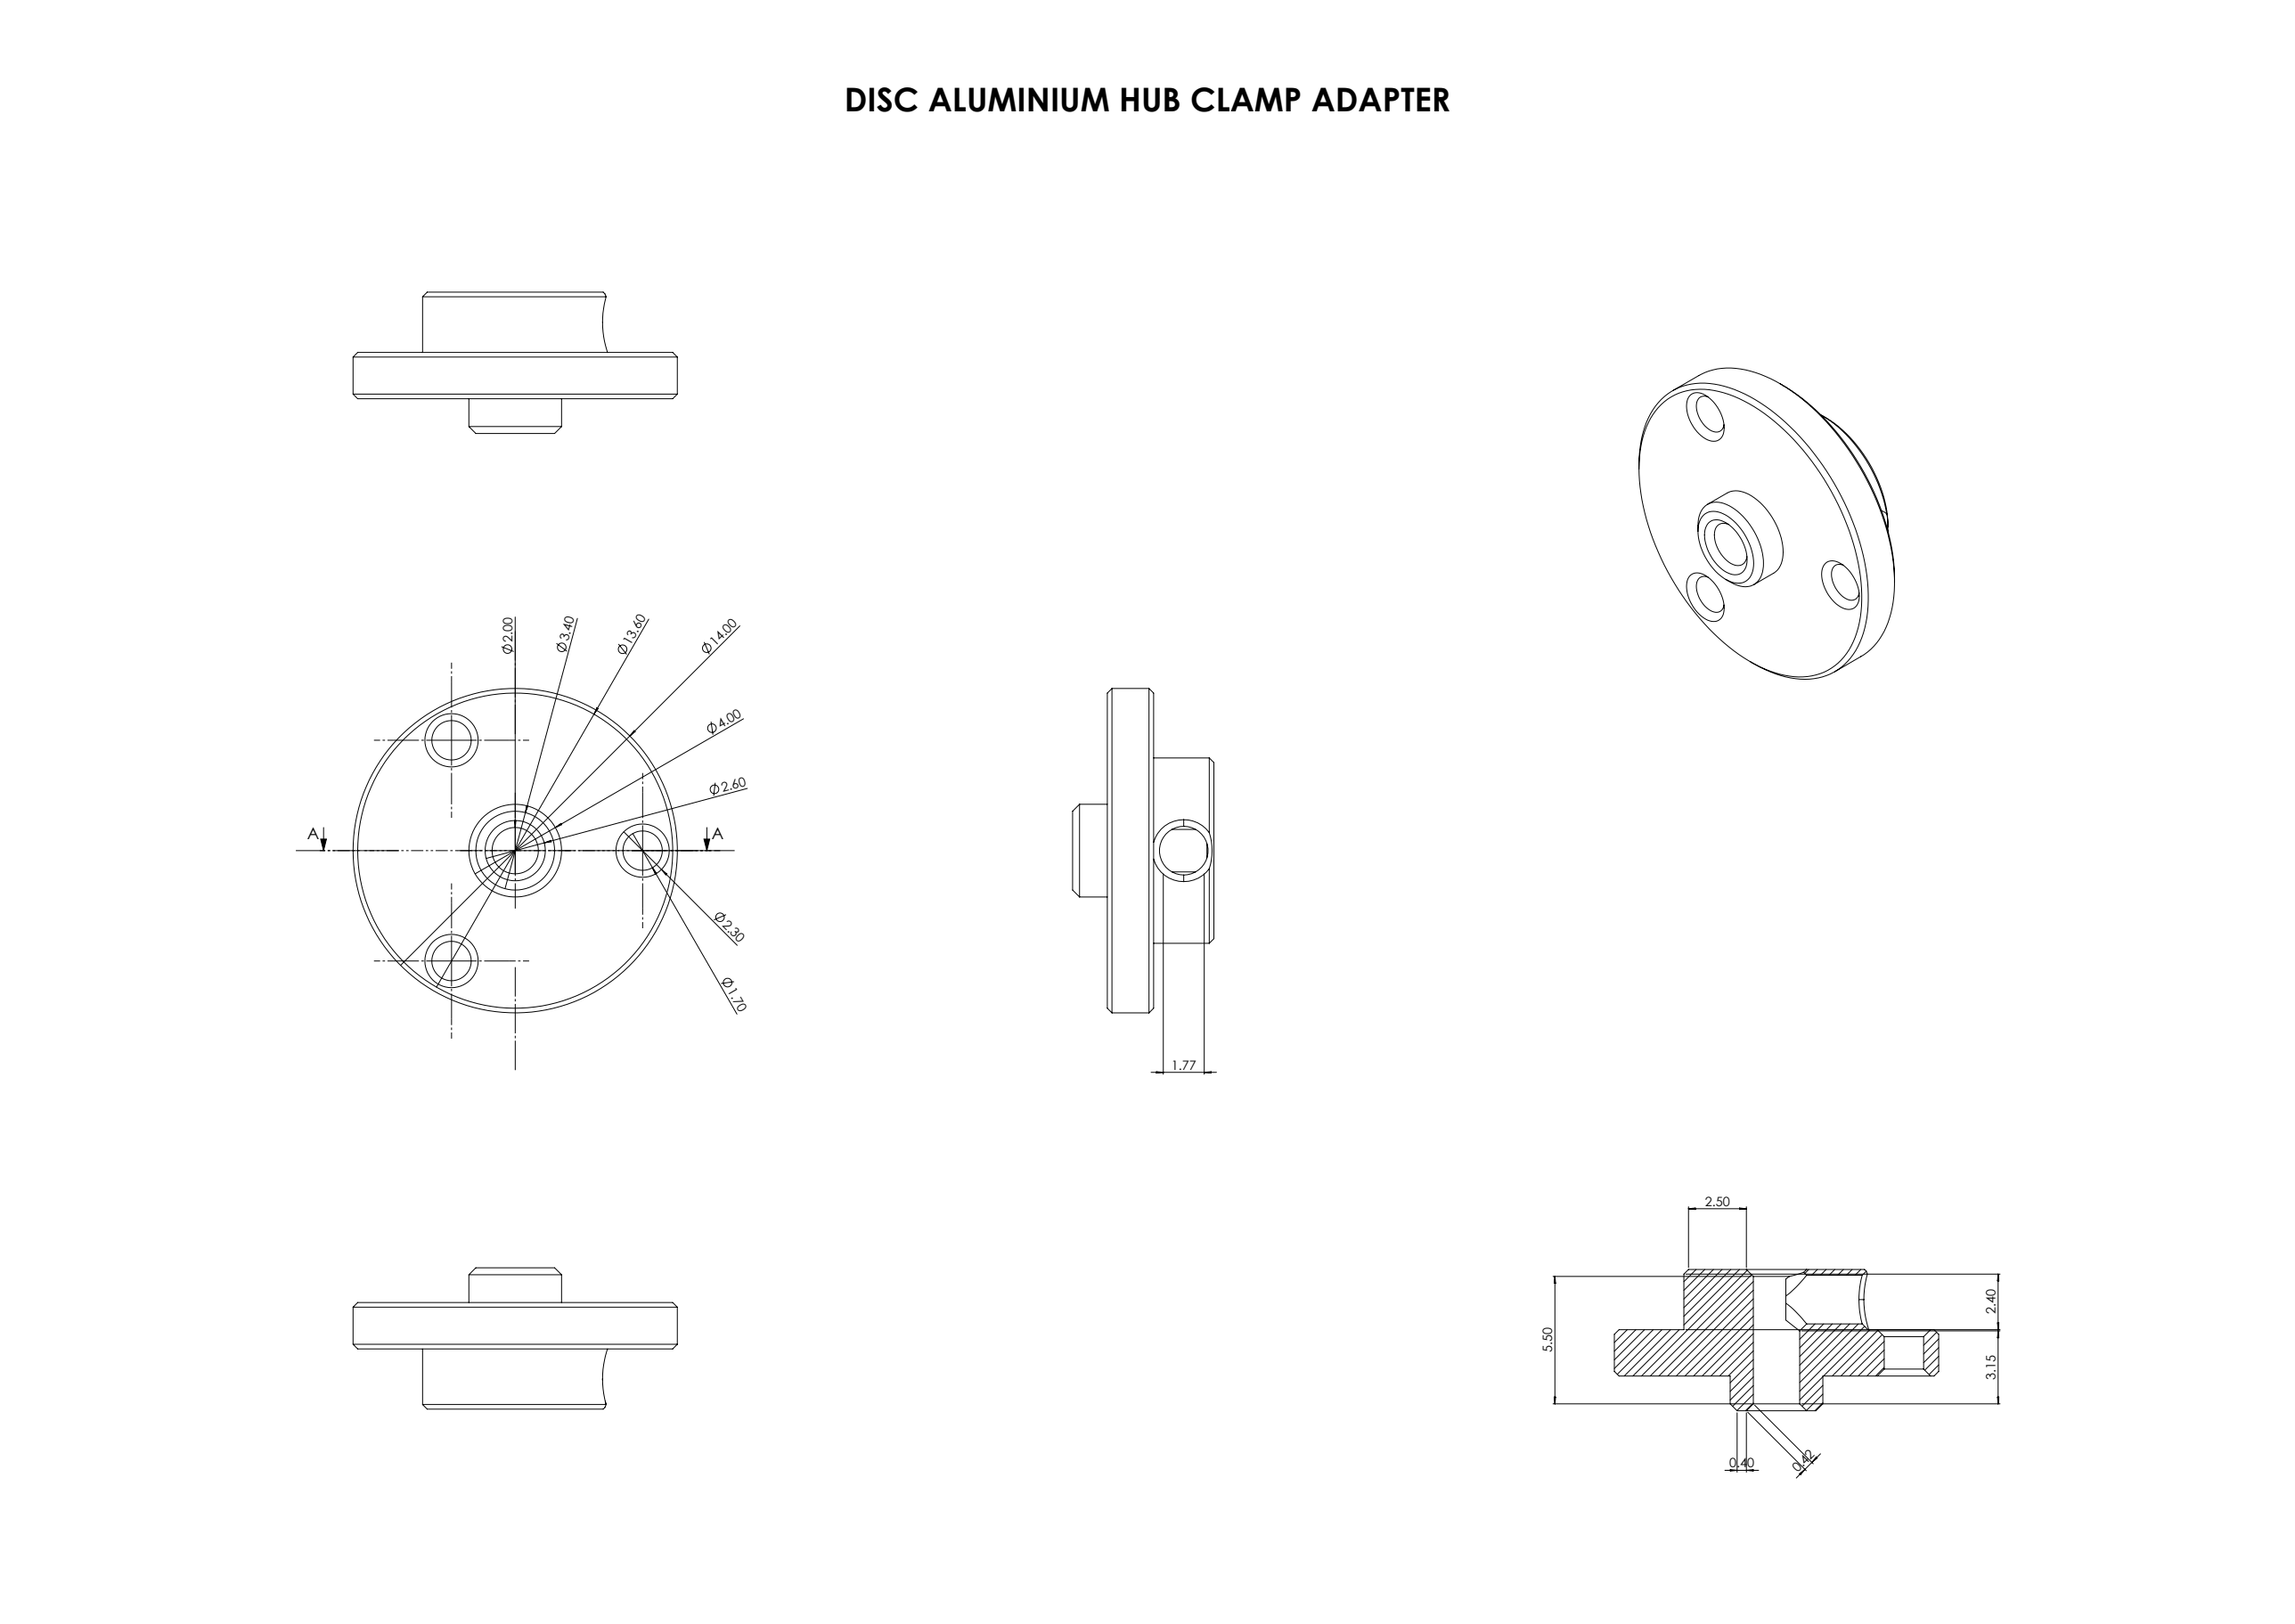
ISO-10303-21;
HEADER;
/* Generated by software containing ST-Developer
 * from STEP Tools, Inc. (www.steptools.com) 
 */

FILE_DESCRIPTION(
/* description */ (''),
/* implementation_level */ '2;1');

FILE_NAME(
/* name */ '08_Disc_Aluminium_Hub_Clamp_Adapter.step',
/* time_stamp */ '2026-10-19T23:00:43-07:00',
/* author */ (''),
/* organization */ (''),
/* preprocessor_version */ 'ST-DEVELOPER v20.2',
/* originating_system */ 'Autodesk Translation Framework v15.15.0.0',
/* authorisation */ '');

FILE_SCHEMA (('AUTOMOTIVE_DESIGN { 1 0 10303 214 3 1 1 }'));
ENDSEC;

DATA;
#10=MECHANICAL_DESIGN_GEOMETRIC_PRESENTATION_REPRESENTATION('',(#1003),#55002);
#467=B_SPLINE_SURFACE_WITH_KNOTS('',3,3,((#36405,#36406,#36407,#36408,#36409,
#36410,#36411,#36412,#36413,#36414,#36415,#36416,#36417,#36418,#36419,#36420,
#36421),(#36422,#36423,#36424,#36425,#36426,#36427,#36428,#36429,#36430,
#36431,#36432,#36433,#36434,#36435,#36436,#36437,#36438),(#36439,#36440,
#36441,#36442,#36443,#36444,#36445,#36446,#36447,#36448,#36449,#36450,#36451,
#36452,#36453,#36454,#36455),(#36456,#36457,#36458,#36459,#36460,#36461,
#36462,#36463,#36464,#36465,#36466,#36467,#36468,#36469,#36470,#36471,#36472)),
 .UNSPECIFIED.,.F.,.F.,.F.,(4,4),(4,2,2,2,1,2,2,2,4),(0.,1.),(0.0282690113416936,
0.0484109685685348,0.093261745053174,0.134172257639861,0.175082770226548,
0.215993282813234,0.256903795399921,0.30175457188456,0.321896529111401),
 .UNSPECIFIED.);
#468=B_SPLINE_SURFACE_WITH_KNOTS('',3,3,((#36507,#36508,#36509,#36510,#36511,
#36512,#36513,#36514,#36515,#36516,#36517,#36518,#36519,#36520,#36521,#36522,
#36523,#36524,#36525,#36526,#36527,#36528,#36529,#36530,#36531,#36532,#36533,
#36534,#36535,#36536,#36537,#36538,#36539,#36540),(#36541,#36542,#36543,
#36544,#36545,#36546,#36547,#36548,#36549,#36550,#36551,#36552,#36553,#36554,
#36555,#36556,#36557,#36558,#36559,#36560,#36561,#36562,#36563,#36564,#36565,
#36566,#36567,#36568,#36569,#36570,#36571,#36572,#36573,#36574),(#36575,
#36576,#36577,#36578,#36579,#36580,#36581,#36582,#36583,#36584,#36585,#36586,
#36587,#36588,#36589,#36590,#36591,#36592,#36593,#36594,#36595,#36596,#36597,
#36598,#36599,#36600,#36601,#36602,#36603,#36604,#36605,#36606,#36607,#36608),
(#36609,#36610,#36611,#36612,#36613,#36614,#36615,#36616,#36617,#36618,
#36619,#36620,#36621,#36622,#36623,#36624,#36625,#36626,#36627,#36628,#36629,
#36630,#36631,#36632,#36633,#36634,#36635,#36636,#36637,#36638,#36639,#36640,
#36641,#36642)),.UNSPECIFIED.,.F.,.T.,.F.,(4,4),(4,2,2,2,2,2,2,2,2,2,2,
2,2,2,2,2,4),(0.,1.),(0.,0.0397570154954407,0.0795140309908814,0.119264247282177,
0.159014463573472,0.198764679864768,0.238514896156063,0.278271911651504,
0.318028927146944,0.357785942642385,0.397542958137826,0.437293174429121,
0.477043390720416,0.516793607011712,0.556543823303007,0.596300838798448,
0.636057854293889),.UNSPECIFIED.);
#469=B_SPLINE_SURFACE_WITH_KNOTS('',3,3,((#36833,#36834,#36835,#36836,#36837,
#36838,#36839,#36840,#36841,#36842,#36843,#36844,#36845,#36846,#36847,#36848,
#36849),(#36850,#36851,#36852,#36853,#36854,#36855,#36856,#36857,#36858,
#36859,#36860,#36861,#36862,#36863,#36864,#36865,#36866),(#36867,#36868,
#36869,#36870,#36871,#36872,#36873,#36874,#36875,#36876,#36877,#36878,#36879,
#36880,#36881,#36882,#36883),(#36884,#36885,#36886,#36887,#36888,#36889,
#36890,#36891,#36892,#36893,#36894,#36895,#36896,#36897,#36898,#36899,#36900)),
 .UNSPECIFIED.,.F.,.F.,.F.,(4,4),(4,2,2,2,1,2,2,2,4),(0.,1.),(0.378434551794792,
0.39857650902163,0.443427285506269,0.484337798092956,0.525248310679643,
0.566158823266329,0.607069335853016,0.651920112337657,0.672062069564494),
 .UNSPECIFIED.);
#486=B_SPLINE_CURVE_WITH_KNOTS('',3,(#36316,#36317,#36318,#36319),
 .UNSPECIFIED.,.F.,.F.,(4,4),(-0.280466891366677,-0.261609752320044),
 .UNSPECIFIED.);
#487=B_SPLINE_CURVE_WITH_KNOTS('',3,(#36323,#36324,#36325,#36326,#36327,
#36328,#36329,#36330,#36331,#36332,#36333,#36334,#36335,#36336,#36337,#36338,
#36339,#36340,#36341,#36342,#36343,#36344,#36345,#36346,#36347,#36348,#36349,
#36350,#36351,#36352,#36353,#36354,#36355,#36356,#36357,#36358,#36359,#36360,
#36361,#36362,#36363,#36364,#36365),.UNSPECIFIED.,.F.,.F.,(4,3,3,3,3,3,
3,3,3,3,3,3,3,3,4),(-0.630634535346295,-0.607069335853016,-0.607059843804484,
-0.566158823266329,-0.566157090505946,-0.545703566972986,-0.530072037367157,
-0.525248310679643,-0.509616781073714,-0.504793054386299,-0.484339530853349,
-0.484337798092956,-0.443436777554782,-0.443427285506269,-0.41986208601299),
 .UNSPECIFIED.);
#488=B_SPLINE_CURVE_WITH_KNOTS('',3,(#36369,#36370,#36371,#36372),
 .UNSPECIFIED.,.F.,.F.,(4,4),(-0.0885671277154287,-0.0696965455598956),
 .UNSPECIFIED.);
#489=B_SPLINE_CURVE_WITH_KNOTS('',3,(#36379,#36380,#36381,#36382,#36383,
#36384,#36385,#36386,#36387,#36388,#36389,#36390),.UNSPECIFIED.,.F.,.F.,
(4,2,2,2,2,4),(-0.113003243228151,-0.107933555890422,-0.0982851988970644,
-0.0760068744412316,-0.0436115274099374,0.),.UNSPECIFIED.);
#490=B_SPLINE_CURVE_WITH_KNOTS('',3,(#36391,#36392,#36393,#36394,#36395,
#36396,#36397,#36398,#36399,#36400,#36401,#36402,#36403,#36404),
 .UNSPECIFIED.,.F.,.F.,(4,2,2,2,2,2,4),(-0.226033312565039,-0.202158826238804,
-0.175315276513873,-0.140039287867993,-0.124092119684883,-0.115509828763379,
-0.113003243228151),.UNSPECIFIED.);
#491=B_SPLINE_CURVE_WITH_KNOTS('',3,(#36474,#36475,#36476,#36477,#36478,
#36479),.UNSPECIFIED.,.F.,.F.,(4,2,4),(0.,0.0362094892516395,0.0734296059630077),
 .UNSPECIFIED.);
#492=B_SPLINE_CURVE_WITH_KNOTS('',3,(#36481,#36482,#36483,#36484,#36485,
#36486,#36487,#36488,#36489,#36490,#36491,#36492,#36493,#36494,#36495,#36496,
#36497),.UNSPECIFIED.,.F.,.F.,(4,2,2,2,1,2,2,2,4),(0.0282690113416936,0.0484109685685348,
0.093261745053174,0.134172257639861,0.175082770226548,0.215993282813234,
0.256903795399921,0.30175457188456,0.321896529111401),.UNSPECIFIED.);
#493=B_SPLINE_CURVE_WITH_KNOTS('',3,(#36498,#36499,#36500,#36501,#36502,
#36503),.UNSPECIFIED.,.F.,.F.,(4,2,4),(0.,0.0226390736381346,0.0740951944294503),
 .UNSPECIFIED.);
#494=B_SPLINE_CURVE_WITH_KNOTS('',3,(#36645,#36646,#36647,#36648,#36649,
#36650,#36651,#36652,#36653,#36654,#36655,#36656,#36657,#36658,#36659,#36660,
#36661,#36662,#36663,#36664,#36665,#36666),.UNSPECIFIED.,.F.,.F.,(4,3,3,
3,3,3,3,4),(0.,0.0219501236857843,0.0311547049411958,0.0514821946010744,
0.0630509139948673,0.0721978608080179,0.0771276015421864,0.0795991465120393),
 .UNSPECIFIED.);
#495=B_SPLINE_CURVE_WITH_KNOTS('',3,(#36668,#36669,#36670,#36671,#36672,
#36673,#36674,#36675,#36676,#36677,#36678,#36679,#36680,#36681,#36682,#36683,
#36684,#36685,#36686,#36687,#36688,#36689,#36690,#36691,#36692),
 .UNSPECIFIED.,.F.,.F.,(4,3,3,3,3,3,3,3,4),(0.0795991465120393,0.0812132933260193,
0.0858207670056381,0.0934958456969542,0.108889996793442,0.128005586672169,
0.13522501814088,0.156399787118725,0.15916082106724),.UNSPECIFIED.);
#496=B_SPLINE_CURVE_WITH_KNOTS('',3,(#36694,#36695,#36696,#36697,#36698,
#36699,#36700,#36701),.UNSPECIFIED.,.F.,.F.,(4,2,2,4),(-0.0966517478861538,
-0.0795140309908814,-0.0397570154954407,0.),.UNSPECIFIED.);
#497=B_SPLINE_CURVE_WITH_KNOTS('',3,(#36705,#36706,#36707,#36708,#36709,
#36710,#36711,#36712,#36713,#36714,#36715,#36716,#36717,#36718,#36719,#36720,
#36721,#36722),.UNSPECIFIED.,.F.,.F.,(4,2,2,2,2,2,2,2,4),(0.,0.0397570154954407,
0.0795140309908814,0.119264247282177,0.159014463573472,0.198764679864768,
0.238514896156063,0.278271911651504,0.318028927146944),.UNSPECIFIED.);
#498=B_SPLINE_CURVE_WITH_KNOTS('',3,(#36723,#36724,#36725,#36726,#36727,
#36728,#36729,#36730,#36731,#36732,#36733,#36734,#36735,#36736,#36737,#36738,
#36739,#36740),.UNSPECIFIED.,.F.,.F.,(4,2,2,2,2,2,2,2,4),(0.318028927146944,
0.357785942642385,0.397542958137826,0.437293174429121,0.477043390720416,
0.516793607011712,0.556543823303007,0.596300838798448,0.636057854293889),
 .UNSPECIFIED.);
#499=B_SPLINE_CURVE_WITH_KNOTS('',3,(#36742,#36743,#36744,#36745,#36746,
#36747,#36748,#36749,#36750,#36751),.UNSPECIFIED.,.F.,.F.,(4,2,2,2,4),(-0.636057854293889,
-0.596300838798448,-0.556543823303007,-0.516793607011712,-0.50481556113779),
 .UNSPECIFIED.);
#500=B_SPLINE_CURVE_WITH_KNOTS('',3,(#36753,#36754,#36755,#36756,#36757,
#36758,#36759,#36760,#36761,#36762,#36763,#36764,#36765,#36766,#36767,#36768,
#36769,#36770,#36771,#36772,#36773,#36774,#36775,#36776,#36777,#36778,#36779,
#36780,#36781,#36782,#36783,#36784,#36785,#36786),.UNSPECIFIED.,.F.,.F.,
(4,3,3,3,3,3,3,3,3,3,3,4),(0.,0.0113828656482154,0.0288034752669669,0.0331384756330993,
0.0355386446508756,0.0366033865449319,0.0375600712478615,0.0399178311655261,
0.0440602794471665,0.0525575068012412,0.0713574218751575,0.0732127853373217),
 .UNSPECIFIED.);
#501=B_SPLINE_CURVE_WITH_KNOTS('',3,(#36787,#36788,#36789,#36790,#36791,
#36792,#36793,#36794,#36795,#36796,#36797,#36798,#36799,#36800,#36801,#36802),
 .UNSPECIFIED.,.F.,.F.,(4,2,2,2,2,2,2,4),(-0.449271220303512,-0.437293174429121,
-0.397542958137826,-0.357785942642385,-0.318028927146944,-0.278271911651504,
-0.238514896156063,-0.221377182278887),.UNSPECIFIED.);
#502=B_SPLINE_CURVE_WITH_KNOTS('',3,(#36811,#36812,#36813,#36814,#36815,
#36816,#36817,#36818,#36819,#36820,#36821,#36822,#36823,#36824,#36825,#36826,
#36827),.UNSPECIFIED.,.F.,.F.,(4,2,2,2,1,2,2,2,4),(0.378434551794792,0.39857650902163,
0.443427285506269,0.484337798092956,0.525248310679643,0.566158823266329,
0.607069335853016,0.651920112337657,0.672062069564494),.UNSPECIFIED.);
#503=B_SPLINE_CURVE_WITH_KNOTS('',3,(#36901,#36902,#36903,#36904,#36905,
#36906),.UNSPECIFIED.,.F.,.F.,(4,2,4),(0.,0.0362094557981297,0.0734296064948461),
 .UNSPECIFIED.);
#504=B_SPLINE_CURVE_WITH_KNOTS('',3,(#36907,#36908,#36909,#36910,#36911,
#36912),.UNSPECIFIED.,.F.,.F.,(4,2,4),(0.,0.0226438889259442,0.0740951100387875),
 .UNSPECIFIED.);
#963=SHAPE_REPRESENTATION_RELATIONSHIP('SRR','None',#55111,#983);
#983=ADVANCED_BREP_SHAPE_REPRESENTATION('',(#1023),#54989);
#1003=STYLED_ITEM('',(#55372),#1023);
#1023=MANIFOLD_SOLID_BREP('Hub Clamp Adapter',#24536);
#1197=FACE_BOUND('',#4447,.T.);
#1198=FACE_BOUND('',#4454,.T.);
#1199=FACE_BOUND('',#4463,.T.);
#1200=FACE_BOUND('',#4464,.T.);
#1201=FACE_BOUND('',#4465,.T.);
#1202=FACE_BOUND('',#4466,.T.);
#1203=FACE_BOUND('',#4469,.T.);
#1204=FACE_BOUND('',#4470,.T.);
#1205=FACE_BOUND('',#4471,.T.);
#1206=FACE_BOUND('',#4472,.T.);
#1433=PLANE('',#25850);
#1434=PLANE('',#25862);
#1435=PLANE('',#25877);
#1436=PLANE('',#25883);
#1437=PLANE('',#25897);
#1438=PLANE('',#25898);
#2148=CYLINDRICAL_SURFACE('',#25852,0.2);
#2149=CYLINDRICAL_SURFACE('',#25857,0.1);
#2150=CYLINDRICAL_SURFACE('',#25864,0.4);
#2151=CYLINDRICAL_SURFACE('',#25868,0.105);
#2152=CYLINDRICAL_SURFACE('',#25875,0.085);
#2153=CYLINDRICAL_SURFACE('',#25889,0.085);
#2154=CYLINDRICAL_SURFACE('',#25894,0.085);
#2155=CYLINDRICAL_SURFACE('',#25902,0.7);
#2920=FACE_OUTER_BOUND('',#4445,.T.);
#2921=FACE_OUTER_BOUND('',#4446,.T.);
#2922=FACE_OUTER_BOUND('',#4448,.T.);
#2923=FACE_OUTER_BOUND('',#4449,.T.);
#2924=FACE_OUTER_BOUND('',#4450,.T.);
#2925=FACE_OUTER_BOUND('',#4451,.T.);
#2926=FACE_OUTER_BOUND('',#4452,.T.);
#2927=FACE_OUTER_BOUND('',#4453,.T.);
#2928=FACE_OUTER_BOUND('',#4455,.T.);
#2929=FACE_OUTER_BOUND('',#4456,.T.);
#2930=FACE_OUTER_BOUND('',#4457,.T.);
#2931=FACE_OUTER_BOUND('',#4458,.T.);
#2932=FACE_OUTER_BOUND('',#4459,.T.);
#2933=FACE_OUTER_BOUND('',#4460,.T.);
#2934=FACE_OUTER_BOUND('',#4461,.T.);
#2935=FACE_OUTER_BOUND('',#4462,.T.);
#2936=FACE_OUTER_BOUND('',#4467,.T.);
#2937=FACE_OUTER_BOUND('',#4468,.T.);
#2938=FACE_OUTER_BOUND('',#4473,.T.);
#2939=FACE_OUTER_BOUND('',#4474,.T.);
#2940=FACE_OUTER_BOUND('',#4475,.T.);
#2941=FACE_OUTER_BOUND('',#4476,.T.);
#2942=FACE_OUTER_BOUND('',#4477,.T.);
#2943=FACE_OUTER_BOUND('',#4478,.T.);
#2944=FACE_OUTER_BOUND('',#4479,.T.);
#2945=FACE_OUTER_BOUND('',#4480,.T.);
#2946=FACE_OUTER_BOUND('',#4481,.T.);
#2947=FACE_OUTER_BOUND('',#4482,.T.);
#2948=FACE_OUTER_BOUND('',#4483,.T.);
#4445=EDGE_LOOP('',(#18174,#18175,#18176,#18177,#18178));
#4446=EDGE_LOOP('',(#18179));
#4447=EDGE_LOOP('',(#18180));
#4448=EDGE_LOOP('',(#18181,#18182,#18183,#18184,#18185));
#4449=EDGE_LOOP('',(#18186,#18187,#18188,#18189,#18190));
#4450=EDGE_LOOP('',(#18191,#18192,#18193,#18194,#18195,#18196,#18197,#18198,
#18199,#18200,#18201));
#4451=EDGE_LOOP('',(#18202,#18203,#18204,#18205,#18206,#18207,#18208));
#4452=EDGE_LOOP('',(#18209,#18210,#18211,#18212,#18213,#18214,#18215));
#4453=EDGE_LOOP('',(#18216));
#4454=EDGE_LOOP('',(#18217));
#4455=EDGE_LOOP('',(#18218,#18219,#18220,#18221,#18222,#18223,#18224,#18225,
#18226,#18227));
#4456=EDGE_LOOP('',(#18228,#18229,#18230,#18231,#18232));
#4457=EDGE_LOOP('',(#18233,#18234,#18235,#18236,#18237,#18238));
#4458=EDGE_LOOP('',(#18239,#18240,#18241,#18242,#18243,#18244,#18245,#18246,
#18247));
#4459=EDGE_LOOP('',(#18248,#18249,#18250,#18251));
#4460=EDGE_LOOP('',(#18252,#18253,#18254,#18255));
#4461=EDGE_LOOP('',(#18256,#18257,#18258,#18259));
#4462=EDGE_LOOP('',(#18260));
#4463=EDGE_LOOP('',(#18261));
#4464=EDGE_LOOP('',(#18262,#18263));
#4465=EDGE_LOOP('',(#18264));
#4466=EDGE_LOOP('',(#18265));
#4467=EDGE_LOOP('',(#18266,#18267,#18268,#18269));
#4468=EDGE_LOOP('',(#18270));
#4469=EDGE_LOOP('',(#18271));
#4470=EDGE_LOOP('',(#18272));
#4471=EDGE_LOOP('',(#18273));
#4472=EDGE_LOOP('',(#18274));
#4473=EDGE_LOOP('',(#18275,#18276,#18277,#18278));
#4474=EDGE_LOOP('',(#18279,#18280,#18281,#18282));
#4475=EDGE_LOOP('',(#18283,#18284,#18285,#18286));
#4476=EDGE_LOOP('',(#18287,#18288,#18289,#18290));
#4477=EDGE_LOOP('',(#18291,#18292,#18293,#18294));
#4478=EDGE_LOOP('',(#18295,#18296,#18297,#18298));
#4479=EDGE_LOOP('',(#18299,#18300,#18301,#18302,#18303));
#4480=EDGE_LOOP('',(#18304,#18305,#18306,#18307));
#4481=EDGE_LOOP('',(#18308,#18309,#18310,#18311,#18312));
#4482=EDGE_LOOP('',(#18313,#18314,#18315,#18316,#18317,#18318));
#4483=EDGE_LOOP('',(#18319,#18320,#18321,#18322,#18323));
#5963=LINE('',#36293,#7784);
#5964=LINE('',#36302,#7785);
#5965=LINE('',#36309,#7786);
#5966=LINE('',#36312,#7787);
#5967=LINE('',#36321,#7788);
#5968=LINE('',#36367,#7789);
#5969=LINE('',#36378,#7790);
#5970=LINE('',#36703,#7791);
#5971=LINE('',#36807,#7792);
#5972=LINE('',#36831,#7793);
#5973=LINE('',#36917,#7794);
#5974=LINE('',#36921,#7795);
#5975=LINE('',#36933,#7796);
#5976=LINE('',#36943,#7797);
#5977=LINE('',#36947,#7798);
#5978=LINE('',#36950,#7799);
#5979=LINE('',#36953,#7800);
#5980=LINE('',#36957,#7801);
#5981=LINE('',#36960,#7802);
#5982=LINE('',#36965,#7803);
#5983=LINE('',#36971,#7804);
#5984=LINE('',#36976,#7805);
#7784=VECTOR('',#29935,0.185);
#7785=VECTOR('',#29946,0.2);
#7786=VECTOR('',#29955,0.115);
#7787=VECTOR('',#29958,0.1);
#7788=VECTOR('',#29961,1.);
#7789=VECTOR('',#29962,1.);
#7790=VECTOR('',#29969,0.115);
#7791=VECTOR('',#29974,1.);
#7792=VECTOR('',#29983,0.39);
#7793=VECTOR('',#29990,0.105);
#7794=VECTOR('',#29997,0.1);
#7795=VECTOR('',#30002,0.085);
#7796=VECTOR('',#30017,0.1);
#7797=VECTOR('',#30028,0.1);
#7798=VECTOR('',#30033,0.085);
#7799=VECTOR('',#30038,0.1);
#7800=VECTOR('',#30041,0.1);
#7801=VECTOR('',#30046,0.085);
#7802=VECTOR('',#30051,0.1);
#7803=VECTOR('',#30058,0.69);
#7804=VECTOR('',#30065,0.7);
#7805=VECTOR('',#30072,0.69);
#9581=CIRCLE('',#25847,0.17);
#9582=CIRCLE('',#25848,0.2);
#9583=CIRCLE('',#25849,0.2);
#9584=CIRCLE('',#25851,0.13);
#9585=CIRCLE('',#25853,0.2);
#9586=CIRCLE('',#25855,0.1);
#9587=CIRCLE('',#25856,0.1);
#9588=CIRCLE('',#25858,0.1);
#9589=CIRCLE('',#25859,0.1);
#9590=CIRCLE('',#25861,0.13);
#9591=CIRCLE('',#25863,0.38);
#9592=CIRCLE('',#25865,0.4);
#9593=CIRCLE('',#25866,0.4);
#9594=CIRCLE('',#25869,0.105);
#9595=CIRCLE('',#25870,0.105);
#9596=CIRCLE('',#25871,0.105);
#9597=CIRCLE('',#25873,0.115);
#9598=CIRCLE('',#25874,0.085);
#9599=CIRCLE('',#25876,0.085);
#9600=CIRCLE('',#25878,0.68);
#9601=CIRCLE('',#25879,0.115);
#9602=CIRCLE('',#25880,0.115);
#9603=CIRCLE('',#25882,0.115);
#9604=CIRCLE('',#25884,0.68);
#9605=CIRCLE('',#25885,0.115);
#9606=CIRCLE('',#25886,0.115);
#9607=CIRCLE('',#25888,0.085);
#9608=CIRCLE('',#25890,0.085);
#9609=CIRCLE('',#25893,0.085);
#9610=CIRCLE('',#25895,0.085);
#9611=CIRCLE('',#25900,0.7);
#9612=CIRCLE('',#25901,0.7);
#9613=CIRCLE('',#25903,0.7);
#9614=CIRCLE('',#25904,0.7);
#10767=VERTEX_POINT('',#36290);
#10768=VERTEX_POINT('',#36292);
#10769=VERTEX_POINT('',#36294);
#10770=VERTEX_POINT('',#36298);
#10771=VERTEX_POINT('',#36301);
#10772=VERTEX_POINT('',#36305);
#10773=VERTEX_POINT('',#36306);
#10774=VERTEX_POINT('',#36311);
#10775=VERTEX_POINT('',#36313);
#10776=VERTEX_POINT('',#36315);
#10777=VERTEX_POINT('',#36320);
#10778=VERTEX_POINT('',#36322);
#10779=VERTEX_POINT('',#36366);
#10780=VERTEX_POINT('',#36368);
#10781=VERTEX_POINT('',#36375);
#10782=VERTEX_POINT('',#36377);
#10783=VERTEX_POINT('',#36473);
#10784=VERTEX_POINT('',#36480);
#10785=VERTEX_POINT('',#36505);
#10786=VERTEX_POINT('',#36643);
#10787=VERTEX_POINT('',#36644);
#10788=VERTEX_POINT('',#36667);
#10789=VERTEX_POINT('',#36693);
#10790=VERTEX_POINT('',#36702);
#10791=VERTEX_POINT('',#36704);
#10792=VERTEX_POINT('',#36741);
#10793=VERTEX_POINT('',#36752);
#10794=VERTEX_POINT('',#36809);
#10795=VERTEX_POINT('',#36810);
#10796=VERTEX_POINT('',#36829);
#10797=VERTEX_POINT('',#36914);
#10798=VERTEX_POINT('',#36916);
#10799=VERTEX_POINT('',#36920);
#10800=VERTEX_POINT('',#36924);
#10801=VERTEX_POINT('',#36926);
#10802=VERTEX_POINT('',#36928);
#10803=VERTEX_POINT('',#36931);
#10804=VERTEX_POINT('',#36935);
#10805=VERTEX_POINT('',#36937);
#10806=VERTEX_POINT('',#36939);
#10807=VERTEX_POINT('',#36942);
#10808=VERTEX_POINT('',#36946);
#10809=VERTEX_POINT('',#36952);
#10810=VERTEX_POINT('',#36956);
#10811=VERTEX_POINT('',#36964);
#10812=VERTEX_POINT('',#36966);
#10813=VERTEX_POINT('',#36970);
#10814=VERTEX_POINT('',#36972);
#13495=EDGE_CURVE('',#10767,#10767,#9581,.T.);
#13496=EDGE_CURVE('',#10767,#10768,#5963,.T.);
#13497=EDGE_CURVE('',#10768,#10769,#9582,.T.);
#13498=EDGE_CURVE('',#10769,#10768,#9583,.T.);
#13499=EDGE_CURVE('',#10770,#10770,#9584,.T.);
#13500=EDGE_CURVE('',#10769,#10771,#5964,.T.);
#13501=EDGE_CURVE('',#10771,#10771,#9585,.T.);
#13502=EDGE_CURVE('',#10772,#10773,#9586,.T.);
#13503=EDGE_CURVE('',#10773,#10772,#9587,.T.);
#13504=EDGE_CURVE('',#10772,#10770,#5965,.T.);
#13505=EDGE_CURVE('',#10773,#10774,#5966,.T.);
#13506=EDGE_CURVE('',#10775,#10774,#9588,.T.);
#13507=EDGE_CURVE('',#10776,#10775,#486,.T.);
#13508=EDGE_CURVE('',#10776,#10777,#5967,.T.);
#13509=EDGE_CURVE('',#10778,#10777,#487,.T.);
#13510=EDGE_CURVE('',#10778,#10779,#5968,.T.);
#13511=EDGE_CURVE('',#10780,#10779,#488,.T.);
#13512=EDGE_CURVE('',#10774,#10780,#9589,.T.);
#13513=EDGE_CURVE('',#10781,#10781,#9590,.T.);
#13514=EDGE_CURVE('',#10781,#10782,#5969,.T.);
#13515=EDGE_CURVE('',#10782,#10775,#489,.T.);
#13516=EDGE_CURVE('',#10780,#10782,#490,.T.);
#13517=EDGE_CURVE('',#10779,#10783,#491,.F.);
#13518=EDGE_CURVE('',#10783,#10784,#492,.T.);
#13519=EDGE_CURVE('',#10784,#10776,#493,.F.);
#13520=EDGE_CURVE('',#10785,#10785,#9591,.T.);
#13521=EDGE_CURVE('',#10786,#10787,#494,.T.);
#13522=EDGE_CURVE('',#10787,#10788,#495,.T.);
#13523=EDGE_CURVE('',#10788,#10789,#496,.T.);
#13524=EDGE_CURVE('',#10789,#10790,#5970,.T.);
#13525=EDGE_CURVE('',#10790,#10791,#497,.T.);
#13526=EDGE_CURVE('',#10791,#10790,#498,.T.);
#13527=EDGE_CURVE('',#10789,#10792,#499,.T.);
#13528=EDGE_CURVE('',#10793,#10792,#500,.T.);
#13529=EDGE_CURVE('',#10793,#10786,#501,.T.);
#13530=EDGE_CURVE('',#10786,#10788,#9592,.T.);
#13531=EDGE_CURVE('',#10792,#10793,#9593,.T.);
#13532=EDGE_CURVE('',#10787,#10785,#5971,.T.);
#13533=EDGE_CURVE('',#10794,#10795,#502,.T.);
#13534=EDGE_CURVE('',#10784,#10794,#9594,.T.);
#13535=EDGE_CURVE('',#10796,#10783,#9595,.T.);
#13536=EDGE_CURVE('',#10796,#10791,#5972,.T.);
#13537=EDGE_CURVE('',#10795,#10796,#9596,.T.);
#13538=EDGE_CURVE('',#10777,#10794,#503,.F.);
#13539=EDGE_CURVE('',#10795,#10778,#504,.F.);
#13540=EDGE_CURVE('',#10797,#10797,#9597,.T.);
#13541=EDGE_CURVE('',#10797,#10798,#5973,.T.);
#13542=EDGE_CURVE('',#10798,#10798,#9598,.T.);
#13543=EDGE_CURVE('',#10798,#10799,#5974,.T.);
#13544=EDGE_CURVE('',#10799,#10799,#9599,.T.);
#13545=EDGE_CURVE('',#10800,#10800,#9600,.T.);
#13546=EDGE_CURVE('',#10801,#10801,#9601,.T.);
#13547=EDGE_CURVE('',#10802,#10802,#9602,.T.);
#13548=EDGE_CURVE('',#10803,#10803,#9603,.T.);
#13549=EDGE_CURVE('',#10803,#10799,#5975,.T.);
#13550=EDGE_CURVE('',#10804,#10804,#9604,.T.);
#13551=EDGE_CURVE('',#10805,#10805,#9605,.T.);
#13552=EDGE_CURVE('',#10806,#10806,#9606,.T.);
#13553=EDGE_CURVE('',#10801,#10807,#5976,.T.);
#13554=EDGE_CURVE('',#10807,#10807,#9607,.T.);
#13555=EDGE_CURVE('',#10807,#10808,#5977,.T.);
#13556=EDGE_CURVE('',#10808,#10808,#9608,.T.);
#13557=EDGE_CURVE('',#10805,#10808,#5978,.T.);
#13558=EDGE_CURVE('',#10802,#10809,#5979,.T.);
#13559=EDGE_CURVE('',#10809,#10809,#9609,.T.);
#13560=EDGE_CURVE('',#10809,#10810,#5980,.T.);
#13561=EDGE_CURVE('',#10810,#10810,#9610,.T.);
#13562=EDGE_CURVE('',#10806,#10810,#5981,.T.);
#13563=EDGE_CURVE('',#10804,#10811,#5982,.T.);
#13564=EDGE_CURVE('',#10811,#10812,#9611,.T.);
#13565=EDGE_CURVE('',#10812,#10811,#9612,.T.);
#13566=EDGE_CURVE('',#10812,#10813,#5983,.T.);
#13567=EDGE_CURVE('',#10814,#10813,#9613,.T.);
#13568=EDGE_CURVE('',#10813,#10814,#9614,.T.);
#13569=EDGE_CURVE('',#10814,#10800,#5984,.T.);
#18174=ORIENTED_EDGE('',*,*,#13495,.T.);
#18175=ORIENTED_EDGE('',*,*,#13496,.T.);
#18176=ORIENTED_EDGE('',*,*,#13497,.T.);
#18177=ORIENTED_EDGE('',*,*,#13498,.T.);
#18178=ORIENTED_EDGE('',*,*,#13496,.F.);
#18179=ORIENTED_EDGE('',*,*,#13495,.F.);
#18180=ORIENTED_EDGE('',*,*,#13499,.F.);
#18181=ORIENTED_EDGE('',*,*,#13497,.F.);
#18182=ORIENTED_EDGE('',*,*,#13498,.F.);
#18183=ORIENTED_EDGE('',*,*,#13500,.T.);
#18184=ORIENTED_EDGE('',*,*,#13501,.T.);
#18185=ORIENTED_EDGE('',*,*,#13500,.F.);
#18186=ORIENTED_EDGE('',*,*,#13502,.T.);
#18187=ORIENTED_EDGE('',*,*,#13503,.T.);
#18188=ORIENTED_EDGE('',*,*,#13504,.T.);
#18189=ORIENTED_EDGE('',*,*,#13499,.T.);
#18190=ORIENTED_EDGE('',*,*,#13504,.F.);
#18191=ORIENTED_EDGE('',*,*,#13502,.F.);
#18192=ORIENTED_EDGE('',*,*,#13503,.F.);
#18193=ORIENTED_EDGE('',*,*,#13505,.T.);
#18194=ORIENTED_EDGE('',*,*,#13506,.F.);
#18195=ORIENTED_EDGE('',*,*,#13507,.F.);
#18196=ORIENTED_EDGE('',*,*,#13508,.T.);
#18197=ORIENTED_EDGE('',*,*,#13509,.F.);
#18198=ORIENTED_EDGE('',*,*,#13510,.T.);
#18199=ORIENTED_EDGE('',*,*,#13511,.F.);
#18200=ORIENTED_EDGE('',*,*,#13512,.F.);
#18201=ORIENTED_EDGE('',*,*,#13505,.F.);
#18202=ORIENTED_EDGE('',*,*,#13513,.T.);
#18203=ORIENTED_EDGE('',*,*,#13514,.T.);
#18204=ORIENTED_EDGE('',*,*,#13515,.T.);
#18205=ORIENTED_EDGE('',*,*,#13506,.T.);
#18206=ORIENTED_EDGE('',*,*,#13512,.T.);
#18207=ORIENTED_EDGE('',*,*,#13516,.T.);
#18208=ORIENTED_EDGE('',*,*,#13514,.F.);
#18209=ORIENTED_EDGE('',*,*,#13516,.F.);
#18210=ORIENTED_EDGE('',*,*,#13511,.T.);
#18211=ORIENTED_EDGE('',*,*,#13517,.T.);
#18212=ORIENTED_EDGE('',*,*,#13518,.T.);
#18213=ORIENTED_EDGE('',*,*,#13519,.T.);
#18214=ORIENTED_EDGE('',*,*,#13507,.T.);
#18215=ORIENTED_EDGE('',*,*,#13515,.F.);
#18216=ORIENTED_EDGE('',*,*,#13520,.F.);
#18217=ORIENTED_EDGE('',*,*,#13513,.F.);
#18218=ORIENTED_EDGE('',*,*,#13521,.T.);
#18219=ORIENTED_EDGE('',*,*,#13522,.T.);
#18220=ORIENTED_EDGE('',*,*,#13523,.T.);
#18221=ORIENTED_EDGE('',*,*,#13524,.T.);
#18222=ORIENTED_EDGE('',*,*,#13525,.T.);
#18223=ORIENTED_EDGE('',*,*,#13526,.T.);
#18224=ORIENTED_EDGE('',*,*,#13524,.F.);
#18225=ORIENTED_EDGE('',*,*,#13527,.T.);
#18226=ORIENTED_EDGE('',*,*,#13528,.F.);
#18227=ORIENTED_EDGE('',*,*,#13529,.T.);
#18228=ORIENTED_EDGE('',*,*,#13527,.F.);
#18229=ORIENTED_EDGE('',*,*,#13523,.F.);
#18230=ORIENTED_EDGE('',*,*,#13530,.F.);
#18231=ORIENTED_EDGE('',*,*,#13529,.F.);
#18232=ORIENTED_EDGE('',*,*,#13531,.F.);
#18233=ORIENTED_EDGE('',*,*,#13521,.F.);
#18234=ORIENTED_EDGE('',*,*,#13530,.T.);
#18235=ORIENTED_EDGE('',*,*,#13522,.F.);
#18236=ORIENTED_EDGE('',*,*,#13532,.T.);
#18237=ORIENTED_EDGE('',*,*,#13520,.T.);
#18238=ORIENTED_EDGE('',*,*,#13532,.F.);
#18239=ORIENTED_EDGE('',*,*,#13533,.F.);
#18240=ORIENTED_EDGE('',*,*,#13534,.F.);
#18241=ORIENTED_EDGE('',*,*,#13518,.F.);
#18242=ORIENTED_EDGE('',*,*,#13535,.F.);
#18243=ORIENTED_EDGE('',*,*,#13536,.T.);
#18244=ORIENTED_EDGE('',*,*,#13525,.F.);
#18245=ORIENTED_EDGE('',*,*,#13526,.F.);
#18246=ORIENTED_EDGE('',*,*,#13536,.F.);
#18247=ORIENTED_EDGE('',*,*,#13537,.F.);
#18248=ORIENTED_EDGE('',*,*,#13538,.T.);
#18249=ORIENTED_EDGE('',*,*,#13533,.T.);
#18250=ORIENTED_EDGE('',*,*,#13539,.T.);
#18251=ORIENTED_EDGE('',*,*,#13509,.T.);
#18252=ORIENTED_EDGE('',*,*,#13540,.T.);
#18253=ORIENTED_EDGE('',*,*,#13541,.T.);
#18254=ORIENTED_EDGE('',*,*,#13542,.T.);
#18255=ORIENTED_EDGE('',*,*,#13541,.F.);
#18256=ORIENTED_EDGE('',*,*,#13542,.F.);
#18257=ORIENTED_EDGE('',*,*,#13543,.T.);
#18258=ORIENTED_EDGE('',*,*,#13544,.F.);
#18259=ORIENTED_EDGE('',*,*,#13543,.F.);
#18260=ORIENTED_EDGE('',*,*,#13545,.F.);
#18261=ORIENTED_EDGE('',*,*,#13546,.F.);
#18262=ORIENTED_EDGE('',*,*,#13531,.T.);
#18263=ORIENTED_EDGE('',*,*,#13528,.T.);
#18264=ORIENTED_EDGE('',*,*,#13547,.F.);
#18265=ORIENTED_EDGE('',*,*,#13540,.F.);
#18266=ORIENTED_EDGE('',*,*,#13548,.T.);
#18267=ORIENTED_EDGE('',*,*,#13549,.T.);
#18268=ORIENTED_EDGE('',*,*,#13544,.T.);
#18269=ORIENTED_EDGE('',*,*,#13549,.F.);
#18270=ORIENTED_EDGE('',*,*,#13550,.F.);
#18271=ORIENTED_EDGE('',*,*,#13551,.F.);
#18272=ORIENTED_EDGE('',*,*,#13501,.F.);
#18273=ORIENTED_EDGE('',*,*,#13552,.F.);
#18274=ORIENTED_EDGE('',*,*,#13548,.F.);
#18275=ORIENTED_EDGE('',*,*,#13546,.T.);
#18276=ORIENTED_EDGE('',*,*,#13553,.T.);
#18277=ORIENTED_EDGE('',*,*,#13554,.T.);
#18278=ORIENTED_EDGE('',*,*,#13553,.F.);
#18279=ORIENTED_EDGE('',*,*,#13554,.F.);
#18280=ORIENTED_EDGE('',*,*,#13555,.T.);
#18281=ORIENTED_EDGE('',*,*,#13556,.F.);
#18282=ORIENTED_EDGE('',*,*,#13555,.F.);
#18283=ORIENTED_EDGE('',*,*,#13551,.T.);
#18284=ORIENTED_EDGE('',*,*,#13557,.T.);
#18285=ORIENTED_EDGE('',*,*,#13556,.T.);
#18286=ORIENTED_EDGE('',*,*,#13557,.F.);
#18287=ORIENTED_EDGE('',*,*,#13547,.T.);
#18288=ORIENTED_EDGE('',*,*,#13558,.T.);
#18289=ORIENTED_EDGE('',*,*,#13559,.T.);
#18290=ORIENTED_EDGE('',*,*,#13558,.F.);
#18291=ORIENTED_EDGE('',*,*,#13559,.F.);
#18292=ORIENTED_EDGE('',*,*,#13560,.T.);
#18293=ORIENTED_EDGE('',*,*,#13561,.F.);
#18294=ORIENTED_EDGE('',*,*,#13560,.F.);
#18295=ORIENTED_EDGE('',*,*,#13552,.T.);
#18296=ORIENTED_EDGE('',*,*,#13562,.T.);
#18297=ORIENTED_EDGE('',*,*,#13561,.T.);
#18298=ORIENTED_EDGE('',*,*,#13562,.F.);
#18299=ORIENTED_EDGE('',*,*,#13510,.F.);
#18300=ORIENTED_EDGE('',*,*,#13539,.F.);
#18301=ORIENTED_EDGE('',*,*,#13537,.T.);
#18302=ORIENTED_EDGE('',*,*,#13535,.T.);
#18303=ORIENTED_EDGE('',*,*,#13517,.F.);
#18304=ORIENTED_EDGE('',*,*,#13508,.F.);
#18305=ORIENTED_EDGE('',*,*,#13519,.F.);
#18306=ORIENTED_EDGE('',*,*,#13534,.T.);
#18307=ORIENTED_EDGE('',*,*,#13538,.F.);
#18308=ORIENTED_EDGE('',*,*,#13550,.T.);
#18309=ORIENTED_EDGE('',*,*,#13563,.T.);
#18310=ORIENTED_EDGE('',*,*,#13564,.T.);
#18311=ORIENTED_EDGE('',*,*,#13565,.T.);
#18312=ORIENTED_EDGE('',*,*,#13563,.F.);
#18313=ORIENTED_EDGE('',*,*,#13564,.F.);
#18314=ORIENTED_EDGE('',*,*,#13565,.F.);
#18315=ORIENTED_EDGE('',*,*,#13566,.T.);
#18316=ORIENTED_EDGE('',*,*,#13567,.F.);
#18317=ORIENTED_EDGE('',*,*,#13568,.F.);
#18318=ORIENTED_EDGE('',*,*,#13566,.F.);
#18319=ORIENTED_EDGE('',*,*,#13567,.T.);
#18320=ORIENTED_EDGE('',*,*,#13568,.T.);
#18321=ORIENTED_EDGE('',*,*,#13569,.T.);
#18322=ORIENTED_EDGE('',*,*,#13545,.T.);
#18323=ORIENTED_EDGE('',*,*,#13569,.F.);
#23109=CONICAL_SURFACE('',#25846,0.185,0.785398163397459);
#23110=CONICAL_SURFACE('',#25854,0.115,0.785398163397459);
#23111=CONICAL_SURFACE('',#25860,0.115,0.785398163397459);
#23112=CONICAL_SURFACE('',#25867,0.39,0.785398163397459);
#23113=CONICAL_SURFACE('',#25872,0.1,0.785398163397459);
#23114=CONICAL_SURFACE('',#25881,0.1,0.785398163397459);
#23115=CONICAL_SURFACE('',#25887,0.1,0.785398163397459);
#23116=CONICAL_SURFACE('',#25891,0.1,0.785398163397459);
#23117=CONICAL_SURFACE('',#25892,0.1,0.785398163397459);
#23118=CONICAL_SURFACE('',#25896,0.1,0.785398163397459);
#23119=CONICAL_SURFACE('',#25899,0.69,0.785398163397459);
#23120=CONICAL_SURFACE('',#25905,0.69,0.785398163397459);
#23673=ADVANCED_FACE('',(#2920),#23109,.T.);
#23674=ADVANCED_FACE('',(#2921,#1197),#1433,.T.);
#23675=ADVANCED_FACE('',(#2922),#2148,.T.);
#23676=ADVANCED_FACE('',(#2923),#23110,.F.);
#23677=ADVANCED_FACE('',(#2924),#2149,.F.);
#23678=ADVANCED_FACE('',(#2925),#23111,.F.);
#23679=ADVANCED_FACE('',(#2926),#467,.T.);
#23680=ADVANCED_FACE('',(#2927,#1198),#1434,.T.);
#23681=ADVANCED_FACE('',(#2928),#468,.T.);
#23682=ADVANCED_FACE('',(#2929),#2150,.T.);
#23683=ADVANCED_FACE('',(#2930),#23112,.T.);
#23684=ADVANCED_FACE('',(#2931),#2151,.F.);
#23685=ADVANCED_FACE('',(#2932),#469,.T.);
#23686=ADVANCED_FACE('',(#2933),#23113,.F.);
#23687=ADVANCED_FACE('',(#2934),#2152,.F.);
#23688=ADVANCED_FACE('',(#2935,#1199,#1200,#1201,#1202),#1435,.T.);
#23689=ADVANCED_FACE('',(#2936),#23114,.F.);
#23690=ADVANCED_FACE('',(#2937,#1203,#1204,#1205,#1206),#1436,.T.);
#23691=ADVANCED_FACE('',(#2938),#23115,.F.);
#23692=ADVANCED_FACE('',(#2939),#2153,.F.);
#23693=ADVANCED_FACE('',(#2940),#23116,.F.);
#23694=ADVANCED_FACE('',(#2941),#23117,.F.);
#23695=ADVANCED_FACE('',(#2942),#2154,.F.);
#23696=ADVANCED_FACE('',(#2943),#23118,.F.);
#23697=ADVANCED_FACE('',(#2944),#1437,.F.);
#23698=ADVANCED_FACE('',(#2945),#1438,.F.);
#23699=ADVANCED_FACE('',(#2946),#23119,.T.);
#23700=ADVANCED_FACE('',(#2947),#2155,.T.);
#23701=ADVANCED_FACE('',(#2948),#23120,.T.);
#24536=CLOSED_SHELL('',(#23673,#23674,#23675,#23676,#23677,#23678,#23679,
#23680,#23681,#23682,#23683,#23684,#23685,#23686,#23687,#23688,#23689,#23690,
#23691,#23692,#23693,#23694,#23695,#23696,#23697,#23698,#23699,#23700,#23701));
#25845=AXIS2_PLACEMENT_3D('',#36288,#29929,#29930);
#25846=AXIS2_PLACEMENT_3D('',#36289,#29931,#29932);
#25847=AXIS2_PLACEMENT_3D('',#36291,#29933,#29934);
#25848=AXIS2_PLACEMENT_3D('',#36295,#29936,#29937);
#25849=AXIS2_PLACEMENT_3D('',#36296,#29938,#29939);
#25850=AXIS2_PLACEMENT_3D('',#36297,#29940,#29941);
#25851=AXIS2_PLACEMENT_3D('',#36299,#29942,#29943);
#25852=AXIS2_PLACEMENT_3D('',#36300,#29944,#29945);
#25853=AXIS2_PLACEMENT_3D('',#36303,#29947,#29948);
#25854=AXIS2_PLACEMENT_3D('',#36304,#29949,#29950);
#25855=AXIS2_PLACEMENT_3D('',#36307,#29951,#29952);
#25856=AXIS2_PLACEMENT_3D('',#36308,#29953,#29954);
#25857=AXIS2_PLACEMENT_3D('',#36310,#29956,#29957);
#25858=AXIS2_PLACEMENT_3D('',#36314,#29959,#29960);
#25859=AXIS2_PLACEMENT_3D('',#36373,#29963,#29964);
#25860=AXIS2_PLACEMENT_3D('',#36374,#29965,#29966);
#25861=AXIS2_PLACEMENT_3D('',#36376,#29967,#29968);
#25862=AXIS2_PLACEMENT_3D('',#36504,#29970,#29971);
#25863=AXIS2_PLACEMENT_3D('',#36506,#29972,#29973);
#25864=AXIS2_PLACEMENT_3D('',#36803,#29975,#29976);
#25865=AXIS2_PLACEMENT_3D('',#36804,#29977,#29978);
#25866=AXIS2_PLACEMENT_3D('',#36805,#29979,#29980);
#25867=AXIS2_PLACEMENT_3D('',#36806,#29981,#29982);
#25868=AXIS2_PLACEMENT_3D('',#36808,#29984,#29985);
#25869=AXIS2_PLACEMENT_3D('',#36828,#29986,#29987);
#25870=AXIS2_PLACEMENT_3D('',#36830,#29988,#29989);
#25871=AXIS2_PLACEMENT_3D('',#36832,#29991,#29992);
#25872=AXIS2_PLACEMENT_3D('',#36913,#29993,#29994);
#25873=AXIS2_PLACEMENT_3D('',#36915,#29995,#29996);
#25874=AXIS2_PLACEMENT_3D('',#36918,#29998,#29999);
#25875=AXIS2_PLACEMENT_3D('',#36919,#30000,#30001);
#25876=AXIS2_PLACEMENT_3D('',#36922,#30003,#30004);
#25877=AXIS2_PLACEMENT_3D('',#36923,#30005,#30006);
#25878=AXIS2_PLACEMENT_3D('',#36925,#30007,#30008);
#25879=AXIS2_PLACEMENT_3D('',#36927,#30009,#30010);
#25880=AXIS2_PLACEMENT_3D('',#36929,#30011,#30012);
#25881=AXIS2_PLACEMENT_3D('',#36930,#30013,#30014);
#25882=AXIS2_PLACEMENT_3D('',#36932,#30015,#30016);
#25883=AXIS2_PLACEMENT_3D('',#36934,#30018,#30019);
#25884=AXIS2_PLACEMENT_3D('',#36936,#30020,#30021);
#25885=AXIS2_PLACEMENT_3D('',#36938,#30022,#30023);
#25886=AXIS2_PLACEMENT_3D('',#36940,#30024,#30025);
#25887=AXIS2_PLACEMENT_3D('',#36941,#30026,#30027);
#25888=AXIS2_PLACEMENT_3D('',#36944,#30029,#30030);
#25889=AXIS2_PLACEMENT_3D('',#36945,#30031,#30032);
#25890=AXIS2_PLACEMENT_3D('',#36948,#30034,#30035);
#25891=AXIS2_PLACEMENT_3D('',#36949,#30036,#30037);
#25892=AXIS2_PLACEMENT_3D('',#36951,#30039,#30040);
#25893=AXIS2_PLACEMENT_3D('',#36954,#30042,#30043);
#25894=AXIS2_PLACEMENT_3D('',#36955,#30044,#30045);
#25895=AXIS2_PLACEMENT_3D('',#36958,#30047,#30048);
#25896=AXIS2_PLACEMENT_3D('',#36959,#30049,#30050);
#25897=AXIS2_PLACEMENT_3D('',#36961,#30052,#30053);
#25898=AXIS2_PLACEMENT_3D('',#36962,#30054,#30055);
#25899=AXIS2_PLACEMENT_3D('',#36963,#30056,#30057);
#25900=AXIS2_PLACEMENT_3D('',#36967,#30059,#30060);
#25901=AXIS2_PLACEMENT_3D('',#36968,#30061,#30062);
#25902=AXIS2_PLACEMENT_3D('',#36969,#30063,#30064);
#25903=AXIS2_PLACEMENT_3D('',#36973,#30066,#30067);
#25904=AXIS2_PLACEMENT_3D('',#36974,#30068,#30069);
#25905=AXIS2_PLACEMENT_3D('',#36975,#30070,#30071);
#29929=DIRECTION('axis',(0.,0.,1.));
#29930=DIRECTION('refdir',(1.,0.,0.));
#29931=DIRECTION('center_axis',(0.,0.,-1.));
#29932=DIRECTION('ref_axis',(-1.,0.,0.));
#29933=DIRECTION('center_axis',(0.,0.,-1.));
#29934=DIRECTION('ref_axis',(-1.,0.,0.));
#29935=DIRECTION('',(0.707106781186555,8.65956056235503E-17,-0.70710678118654));
#29936=DIRECTION('center_axis',(0.,0.,1.));
#29937=DIRECTION('ref_axis',(-1.,0.,0.));
#29938=DIRECTION('center_axis',(0.,0.,1.));
#29939=DIRECTION('ref_axis',(-1.,0.,0.));
#29940=DIRECTION('center_axis',(0.,0.,1.));
#29941=DIRECTION('ref_axis',(1.,0.,0.));
#29942=DIRECTION('center_axis',(0.,0.,1.));
#29943=DIRECTION('ref_axis',(-1.,0.,0.));
#29944=DIRECTION('center_axis',(0.,0.,1.));
#29945=DIRECTION('ref_axis',(1.,0.,0.));
#29946=DIRECTION('',(0.,0.,-1.));
#29947=DIRECTION('center_axis',(0.,0.,1.));
#29948=DIRECTION('ref_axis',(1.,0.,0.));
#29949=DIRECTION('center_axis',(0.,0.,1.));
#29950=DIRECTION('ref_axis',(-1.,0.,0.));
#29951=DIRECTION('center_axis',(0.,0.,-1.));
#29952=DIRECTION('ref_axis',(-1.,0.,0.));
#29953=DIRECTION('center_axis',(0.,0.,-1.));
#29954=DIRECTION('ref_axis',(-1.,0.,0.));
#29955=DIRECTION('',(0.707106781186555,-8.65956056235502E-17,0.70710678118654));
#29956=DIRECTION('center_axis',(0.,0.,1.));
#29957=DIRECTION('ref_axis',(1.,0.,0.));
#29958=DIRECTION('',(0.,0.,-1.));
#29959=DIRECTION('center_axis',(0.,0.,1.));
#29960=DIRECTION('ref_axis',(-1.,0.,0.));
#29961=DIRECTION('',(0.,0.,1.));
#29962=DIRECTION('',(0.,0.,-1.));
#29963=DIRECTION('center_axis',(0.,0.,1.));
#29964=DIRECTION('ref_axis',(-1.,0.,0.));
#29965=DIRECTION('center_axis',(0.,0.,-1.));
#29966=DIRECTION('ref_axis',(-1.,0.,0.));
#29967=DIRECTION('center_axis',(0.,0.,-1.));
#29968=DIRECTION('ref_axis',(-1.,0.,0.));
#29969=DIRECTION('',(-0.707106781186555,8.65956056235503E-17,0.70710678118654));
#29970=DIRECTION('center_axis',(0.,0.,-1.));
#29971=DIRECTION('ref_axis',(-1.,0.,0.));
#29972=DIRECTION('center_axis',(0.,0.,1.));
#29973=DIRECTION('ref_axis',(-1.,0.,0.));
#29974=DIRECTION('',(-0.592241372047889,-0.805760607894698,-4.99896642157306E-14));
#29975=DIRECTION('center_axis',(0.,0.,1.));
#29976=DIRECTION('ref_axis',(-1.,-7.64599154681893E-13,0.));
#29977=DIRECTION('center_axis',(0.,0.,-1.));
#29978=DIRECTION('ref_axis',(-1.,0.,0.));
#29979=DIRECTION('center_axis',(0.,0.,1.));
#29980=DIRECTION('ref_axis',(1.,0.,0.));
#29981=DIRECTION('center_axis',(0.,0.,1.));
#29982=DIRECTION('ref_axis',(-1.,0.,0.));
#29983=DIRECTION('',(-0.707106781186555,-8.65956056235503E-17,-0.70710678118654));
#29984=DIRECTION('center_axis',(1.,0.,0.));
#29985=DIRECTION('ref_axis',(0.,1.,0.));
#29986=DIRECTION('center_axis',(1.,0.,0.));
#29987=DIRECTION('ref_axis',(0.,0.,-1.));
#29988=DIRECTION('center_axis',(1.,0.,0.));
#29989=DIRECTION('ref_axis',(0.,0.,-1.));
#29990=DIRECTION('',(1.,0.,0.));
#29991=DIRECTION('center_axis',(1.,0.,0.));
#29992=DIRECTION('ref_axis',(0.,0.,-1.));
#29993=DIRECTION('center_axis',(0.,0.,-1.));
#29994=DIRECTION('ref_axis',(1.,0.,0.));
#29995=DIRECTION('center_axis',(0.,0.,-1.));
#29996=DIRECTION('ref_axis',(1.,0.,0.));
#29997=DIRECTION('',(0.707106781186555,-8.65956056235503E-17,0.70710678118654));
#29998=DIRECTION('center_axis',(0.,0.,1.));
#29999=DIRECTION('ref_axis',(1.,0.,0.));
#30000=DIRECTION('center_axis',(0.,0.,1.));
#30001=DIRECTION('ref_axis',(1.,0.,0.));
#30002=DIRECTION('',(0.,0.,1.));
#30003=DIRECTION('center_axis',(0.,0.,-1.));
#30004=DIRECTION('ref_axis',(1.,0.,0.));
#30005=DIRECTION('center_axis',(0.,0.,-1.));
#30006=DIRECTION('ref_axis',(-1.,0.,0.));
#30007=DIRECTION('center_axis',(0.,0.,1.));
#30008=DIRECTION('ref_axis',(-1.,0.,0.));
#30009=DIRECTION('center_axis',(0.,0.,-1.));
#30010=DIRECTION('ref_axis',(1.,0.,0.));
#30011=DIRECTION('center_axis',(0.,0.,-1.));
#30012=DIRECTION('ref_axis',(1.,0.,0.));
#30013=DIRECTION('center_axis',(0.,0.,1.));
#30014=DIRECTION('ref_axis',(1.,0.,0.));
#30015=DIRECTION('center_axis',(0.,0.,1.));
#30016=DIRECTION('ref_axis',(1.,0.,0.));
#30017=DIRECTION('',(0.707106781186555,8.65956056235503E-17,-0.70710678118654));
#30018=DIRECTION('center_axis',(0.,0.,1.));
#30019=DIRECTION('ref_axis',(1.,0.,0.));
#30020=DIRECTION('center_axis',(0.,0.,-1.));
#30021=DIRECTION('ref_axis',(-1.,0.,0.));
#30022=DIRECTION('center_axis',(0.,0.,1.));
#30023=DIRECTION('ref_axis',(1.,0.,0.));
#30024=DIRECTION('center_axis',(0.,0.,1.));
#30025=DIRECTION('ref_axis',(1.,0.,0.));
#30026=DIRECTION('center_axis',(0.,0.,-1.));
#30027=DIRECTION('ref_axis',(1.,0.,0.));
#30028=DIRECTION('',(0.707106781186555,-8.65956056235502E-17,0.70710678118654));
#30029=DIRECTION('center_axis',(0.,0.,1.));
#30030=DIRECTION('ref_axis',(1.,0.,0.));
#30031=DIRECTION('center_axis',(0.,0.,1.));
#30032=DIRECTION('ref_axis',(1.,0.,0.));
#30033=DIRECTION('',(0.,0.,1.));
#30034=DIRECTION('center_axis',(0.,0.,-1.));
#30035=DIRECTION('ref_axis',(1.,0.,0.));
#30036=DIRECTION('center_axis',(0.,0.,1.));
#30037=DIRECTION('ref_axis',(1.,0.,0.));
#30038=DIRECTION('',(0.707106781186555,8.65956056235502E-17,-0.70710678118654));
#30039=DIRECTION('center_axis',(0.,0.,-1.));
#30040=DIRECTION('ref_axis',(1.,0.,0.));
#30041=DIRECTION('',(0.707106781186555,-8.65956056235502E-17,0.70710678118654));
#30042=DIRECTION('center_axis',(0.,0.,1.));
#30043=DIRECTION('ref_axis',(1.,0.,0.));
#30044=DIRECTION('center_axis',(0.,0.,1.));
#30045=DIRECTION('ref_axis',(1.,0.,0.));
#30046=DIRECTION('',(0.,0.,1.));
#30047=DIRECTION('center_axis',(0.,0.,-1.));
#30048=DIRECTION('ref_axis',(1.,0.,0.));
#30049=DIRECTION('center_axis',(0.,0.,1.));
#30050=DIRECTION('ref_axis',(1.,0.,0.));
#30051=DIRECTION('',(0.707106781186555,8.65956056235502E-17,-0.70710678118654));
#30052=DIRECTION('center_axis',(-1.,0.,0.));
#30053=DIRECTION('ref_axis',(0.,0.,1.));
#30054=DIRECTION('center_axis',(-1.,0.,0.));
#30055=DIRECTION('ref_axis',(0.,0.,1.));
#30056=DIRECTION('center_axis',(0.,0.,-1.));
#30057=DIRECTION('ref_axis',(-1.,0.,0.));
#30058=DIRECTION('',(0.707106781186555,8.65956056235503E-17,-0.70710678118654));
#30059=DIRECTION('center_axis',(0.,0.,1.));
#30060=DIRECTION('ref_axis',(-1.,0.,0.));
#30061=DIRECTION('center_axis',(0.,0.,1.));
#30062=DIRECTION('ref_axis',(-1.,0.,0.));
#30063=DIRECTION('center_axis',(0.,0.,1.));
#30064=DIRECTION('ref_axis',(1.,0.,0.));
#30065=DIRECTION('',(0.,0.,-1.));
#30066=DIRECTION('center_axis',(0.,0.,-1.));
#30067=DIRECTION('ref_axis',(-1.,0.,0.));
#30068=DIRECTION('center_axis',(0.,0.,-1.));
#30069=DIRECTION('ref_axis',(-1.,0.,0.));
#30070=DIRECTION('center_axis',(0.,0.,1.));
#30071=DIRECTION('ref_axis',(-1.,0.,0.));
#30072=DIRECTION('',(-0.707106781186555,-8.65956056235503E-17,-0.70710678118654));
#36288=CARTESIAN_POINT('',(0.,0.,0.));
#36289=CARTESIAN_POINT('Origin',(0.,0.,11.045));
#36290=CARTESIAN_POINT('',(0.17,-2.0818995585505E-17,11.06));
#36291=CARTESIAN_POINT('Origin',(0.,0.,11.06));
#36292=CARTESIAN_POINT('',(0.2,2.44929359829471E-17,11.03));
#36293=CARTESIAN_POINT('',(0.185,2.2655965784226E-17,11.045));
#36294=CARTESIAN_POINT('',(-0.2,-2.44929359829471E-17,11.03));
#36295=CARTESIAN_POINT('Origin',(0.,0.,11.03));
#36296=CARTESIAN_POINT('Origin',(0.,0.,11.03));
#36297=CARTESIAN_POINT('Origin',(0.1,0.,11.06));
#36298=CARTESIAN_POINT('',(0.13,1.59204083889156E-17,11.06));
#36299=CARTESIAN_POINT('Origin',(0.,0.,11.06));
#36300=CARTESIAN_POINT('Origin',(0.,0.,10.985));
#36301=CARTESIAN_POINT('',(-0.2,-2.44929359829471E-17,10.91));
#36302=CARTESIAN_POINT('',(-0.2,-2.44929359829471E-17,10.985));
#36303=CARTESIAN_POINT('Origin',(0.,0.,10.91));
#36304=CARTESIAN_POINT('Origin',(0.,0.,11.045));
#36305=CARTESIAN_POINT('',(0.1,-1.22464679914735E-17,11.03));
#36306=CARTESIAN_POINT('',(-0.1,-1.22464679914735E-17,11.03));
#36307=CARTESIAN_POINT('Origin',(0.,0.,11.03));
#36308=CARTESIAN_POINT('Origin',(0.,0.,11.03));
#36309=CARTESIAN_POINT('',(0.115,-1.40834381901946E-17,11.045));
#36310=CARTESIAN_POINT('Origin',(0.,0.,10.755));
#36311=CARTESIAN_POINT('',(-0.1,-1.22464679914735E-17,10.48));
#36312=CARTESIAN_POINT('',(-0.1,-1.22464679914735E-17,10.755));
#36313=CARTESIAN_POINT('',(0.0547465096656995,0.0836828517644056,10.48));
#36314=CARTESIAN_POINT('Origin',(0.,0.,10.48));
#36315=CARTESIAN_POINT('',(0.0400022951850117,0.0916331167321948,10.4916905977975));
#36316=CARTESIAN_POINT('Ctrl Pts',(0.0400026971257908,0.091629894956361,
10.4916928986414));
#36317=CARTESIAN_POINT('Ctrl Pts',(0.0449750733872993,0.0894586747527078,
10.4877839912521));
#36318=CARTESIAN_POINT('Ctrl Pts',(0.0499491910902487,0.0868191962733323,
10.4838139809416));
#36319=CARTESIAN_POINT('Ctrl Pts',(0.0547498300911773,0.0836911968368012,
10.4799973371599));
#36320=CARTESIAN_POINT('',(0.0400031709030036,0.091629687702094,10.6683074724692));
#36321=CARTESIAN_POINT('',(0.04,0.0916515138991168,10.755));
#36322=CARTESIAN_POINT('',(0.0400031709030041,-0.0916296877020945,10.6683074724692));
#36323=CARTESIAN_POINT('Ctrl Pts',(0.0400031709030041,-0.0916296877020945,
10.6683074724692));
#36324=CARTESIAN_POINT('Ctrl Pts',(0.0462164496289358,-0.0889165823855752,
10.6731918882274));
#36325=CARTESIAN_POINT('Ctrl Pts',(0.0524198696107662,-0.0854817956373576,
10.6781585108626));
#36326=CARTESIAN_POINT('Ctrl Pts',(0.0583027869865068,-0.0812628967806547,
10.6828213320007));
#36327=CARTESIAN_POINT('Ctrl Pts',(0.0583051566221747,-0.0812611974106702,
10.6828232101823));
#36328=CARTESIAN_POINT('Ctrl Pts',(0.058307526202546,-0.0812594979157138,
10.6828250883107));
#36329=CARTESIAN_POINT('Ctrl Pts',(0.0583098957275982,-0.0812577982957833,
10.682826966386));
#36330=CARTESIAN_POINT('Ctrl Pts',(0.0685201251108097,-0.0739341747962435,
10.6909195499127));
#36331=CARTESIAN_POINT('Ctrl Pts',(0.0791018243371258,-0.0632694863644097,
10.6991954559706));
#36332=CARTESIAN_POINT('Ctrl Pts',(0.0870673985112314,-0.0492439898634108,
10.7052699386598));
#36333=CARTESIAN_POINT('Ctrl Pts',(0.0870677359705705,-0.0492433956771441,
10.7052701960036));
#36334=CARTESIAN_POINT('Ctrl Pts',(0.0870680734252534,-0.049242801484857,
10.7052704533434));
#36335=CARTESIAN_POINT('Ctrl Pts',(0.0870684108752795,-0.0492422072865498,
10.7052707106792));
#36336=CARTESIAN_POINT('Ctrl Pts',(0.0910516748715721,-0.0422282836214033,
10.7083083052616));
#36337=CARTESIAN_POINT('Ctrl Pts',(0.0942888586636921,-0.0343297647086917,
10.7107378284348));
#36338=CARTESIAN_POINT('Ctrl Pts',(0.0965327211088765,-0.0259716063509559,
10.7124125068353));
#36339=CARTESIAN_POINT('Ctrl Pts',(0.0982475846719583,-0.01958391478238,
10.7136923736004));
#36340=CARTESIAN_POINT('Ctrl Pts',(0.0993781637156952,-0.0129130123107152,
10.7145346369017));
#36341=CARTESIAN_POINT('Ctrl Pts',(0.099813360278901,-0.00620869762228023,
10.7148586788687));
#36342=CARTESIAN_POINT('Ctrl Pts',(0.09994765739052,-0.00413981616924315,
10.7149586748335));
#36343=CARTESIAN_POINT('Ctrl Pts',(0.100016017514125,-0.00206780492919306,
10.7150095423241));
#36344=CARTESIAN_POINT('Ctrl Pts',(0.100016017514125,-4.36695016576629E-17,
10.7150095423241));
#36345=CARTESIAN_POINT('Ctrl Pts',(0.100016017514124,0.00670082615866859,
10.7150095423241));
#36346=CARTESIAN_POINT('Ctrl Pts',(0.0992947386787322,0.0134460393231833,
10.7144728477617));
#36347=CARTESIAN_POINT('Ctrl Pts',(0.0979505340509732,0.0199846250780982,
10.713470323343));
#36348=CARTESIAN_POINT('Ctrl Pts',(0.0975357265497413,0.0220023643140571,
10.7131609547838));
#36349=CARTESIAN_POINT('Ctrl Pts',(0.0970619100841739,0.0240004314840473,
10.7128074603445));
#36350=CARTESIAN_POINT('Ctrl Pts',(0.0965327211088716,0.0259716063509535,
10.7124125068353));
#36351=CARTESIAN_POINT('Ctrl Pts',(0.0942888586636877,0.0343297647086844,
10.7107378284348));
#36352=CARTESIAN_POINT('Ctrl Pts',(0.0910516748715695,0.0422282836213917,
10.7083083052616));
#36353=CARTESIAN_POINT('Ctrl Pts',(0.0870684108752762,0.0492422072865391,
10.7052707106792));
#36354=CARTESIAN_POINT('Ctrl Pts',(0.0870680734252483,0.0492428014848496,
10.7052704533434));
#36355=CARTESIAN_POINT('Ctrl Pts',(0.0870677359705637,0.0492433956771398,
10.7052701960036));
#36356=CARTESIAN_POINT('Ctrl Pts',(0.0870673985112227,0.0492439898634097,
10.7052699386598));
#36357=CARTESIAN_POINT('Ctrl Pts',(0.0791018243371071,0.063269486364422,
10.6991954559706));
#36358=CARTESIAN_POINT('Ctrl Pts',(0.0685201251108037,0.0739341747962399,
10.6909195499127));
#36359=CARTESIAN_POINT('Ctrl Pts',(0.0583098957275852,0.0812577982957855,
10.682826966386));
#36360=CARTESIAN_POINT('Ctrl Pts',(0.0583075262025378,0.0812594979157126,
10.6828250883107));
#36361=CARTESIAN_POINT('Ctrl Pts',(0.0583051566221713,0.0812611974106655,
10.6828232101823));
#36362=CARTESIAN_POINT('Ctrl Pts',(0.0583027869865083,0.0812628967806466,
10.6828213320007));
#36363=CARTESIAN_POINT('Ctrl Pts',(0.0524198696107668,0.0854817956373522,
10.6781585108626));
#36364=CARTESIAN_POINT('Ctrl Pts',(0.0462164496289357,0.0889165823855736,
10.6731918882274));
#36365=CARTESIAN_POINT('Ctrl Pts',(0.0400031709030036,0.091629687702094,
10.6683074724692));
#36366=CARTESIAN_POINT('',(0.0400026975908353,-0.0916329430552092,10.4916902797062));
#36367=CARTESIAN_POINT('',(0.04,-0.0916515138991168,10.755));
#36368=CARTESIAN_POINT('',(0.0547465096656977,-0.0836828517644066,10.48));
#36369=CARTESIAN_POINT('Ctrl Pts',(0.0547498564515704,-0.0836911796608913,
10.4799973162027));
#36370=CARTESIAN_POINT('Ctrl Pts',(0.0499493615997624,-0.0868190873748065,
10.4838138453251));
#36371=CARTESIAN_POINT('Ctrl Pts',(0.0449753980973141,-0.0894585033025012,
10.4877837321994));
#36372=CARTESIAN_POINT('Ctrl Pts',(0.0400031703736387,-0.0916296883082219,
10.4916925266094));
#36373=CARTESIAN_POINT('Origin',(0.,0.,10.48));
#36374=CARTESIAN_POINT('Origin',(0.,0.,10.465));
#36375=CARTESIAN_POINT('',(0.13,-1.59204083889156E-17,10.45));
#36376=CARTESIAN_POINT('Origin',(0.,0.,10.45));
#36377=CARTESIAN_POINT('',(0.1175,-5.20790795218413E-18,10.4625));
#36378=CARTESIAN_POINT('',(0.115,-1.40834381901946E-17,10.465));
#36379=CARTESIAN_POINT('Ctrl Pts',(0.1175,3.97378398561307E-18,10.4625));
#36380=CARTESIAN_POINT('Ctrl Pts',(0.1175,0.00168116624611717,10.4625));
#36381=CARTESIAN_POINT('Ctrl Pts',(0.117445299801582,0.00336180897409119,
10.4625186262133));
#36382=CARTESIAN_POINT('Ctrl Pts',(0.11712796129555,0.00823395361238692,
10.4626265875713));
#36383=CARTESIAN_POINT('Ctrl Pts',(0.116722984118053,0.0114065443838321,
10.4627643564121));
#36384=CARTESIAN_POINT('Ctrl Pts',(0.114747805849752,0.0217932663755633,
10.4634333117491));
#36385=CARTESIAN_POINT('Ctrl Pts',(0.112368157615186,0.0287533951010713,
10.4642376426297));
#36386=CARTESIAN_POINT('Ctrl Pts',(0.10440367232782,0.0448544941116708,
10.4668577183297));
#36387=CARTESIAN_POINT('Ctrl Pts',(0.0979725906862171,0.0533246487475542,
10.468932263714));
#36388=CARTESIAN_POINT('Ctrl Pts',(0.0801403078141064,0.0704639960442362,
10.4741919330898));
#36389=CARTESIAN_POINT('Ctrl Pts',(0.0679192198366975,0.0780725887634243,
10.4774832290237));
#36390=CARTESIAN_POINT('Ctrl Pts',(0.0547465096656995,0.0836828517644056,
10.48));
#36391=CARTESIAN_POINT('Ctrl Pts',(0.0547465096656977,-0.0836828517644066,
10.48));
#36392=CARTESIAN_POINT('Ctrl Pts',(0.061953028387731,-0.0806135923009201,
10.4786231263784));
#36393=CARTESIAN_POINT('Ctrl Pts',(0.0688691022940564,-0.0769503000424395,
10.4770113369889));
#36394=CARTESIAN_POINT('Ctrl Pts',(0.0826170742067669,-0.067802259687565,
10.4734642639149));
#36395=CARTESIAN_POINT('Ctrl Pts',(0.0893317161066329,-0.062146954826949,
10.4715149522659));
#36396=CARTESIAN_POINT('Ctrl Pts',(0.102911979968346,-0.0471215719111262,
10.4673741996323));
#36397=CARTESIAN_POINT('Ctrl Pts',(0.109049928744403,-0.0372655563958094,
10.4653399473256));
#36398=CARTESIAN_POINT('Ctrl Pts',(0.11469710309367,-0.0213425122859003,
10.4634512615441));
#36399=CARTESIAN_POINT('Ctrl Pts',(0.115970092871191,-0.0162235405860467,
10.4630196858142));
#36400=CARTESIAN_POINT('Ctrl Pts',(0.117120046050328,-0.00817532652652597,
10.4626293532478));
#36401=CARTESIAN_POINT('Ctrl Pts',(0.117368256214482,-0.00533987258579196,
10.4625448416866));
#36402=CARTESIAN_POINT('Ctrl Pts',(0.117486627839774,-0.0016625527838929,
10.4625045523855));
#36403=CARTESIAN_POINT('Ctrl Pts',(0.1175,-0.000831212403074635,10.4625));
#36404=CARTESIAN_POINT('Ctrl Pts',(0.1175,3.97378398561307E-18,10.4625));
#36405=CARTESIAN_POINT('Ctrl Pts',(0.00894444267269597,-0.0995991814488194,
10.5141610714912));
#36406=CARTESIAN_POINT('Ctrl Pts',(0.0132379567575632,-0.0992136050812441,
10.5116620905429));
#36407=CARTESIAN_POINT('Ctrl Pts',(0.0183531525220914,-0.0984395027524004,
10.5081248887167));
#36408=CARTESIAN_POINT('Ctrl Pts',(0.034707695840997,-0.0945110281336789,
10.4960700069752));
#36409=CARTESIAN_POINT('Ctrl Pts',(0.0471226257755256,-0.0892804815421576,
10.4860357640661));
#36410=CARTESIAN_POINT('Ctrl Pts',(0.0685122634921431,-0.0739398417001646,
10.4690867488427));
#36411=CARTESIAN_POINT('Ctrl Pts',(0.0790926322048203,-0.0632798178846318,
10.4608050384725));
#36412=CARTESIAN_POINT('Ctrl Pts',(0.0950417827106649,-0.0352045502384536,
10.4486511121129));
#36413=CARTESIAN_POINT('Ctrl Pts',(0.10499024921961,2.0497699264001E-14,
10.4413298003685));
#36414=CARTESIAN_POINT('Ctrl Pts',(0.0950417827106623,0.0352045502384679,
10.4486511121129));
#36415=CARTESIAN_POINT('Ctrl Pts',(0.0790926322048192,0.063279817884641,
10.4608050384725));
#36416=CARTESIAN_POINT('Ctrl Pts',(0.0685122634921198,0.0739398417001872,
10.4690867488427));
#36417=CARTESIAN_POINT('Ctrl Pts',(0.0471226257755508,0.0892804815421436,
10.4860357640661));
#36418=CARTESIAN_POINT('Ctrl Pts',(0.0347076958409767,0.0945110281336857,
10.4960700069752));
#36419=CARTESIAN_POINT('Ctrl Pts',(0.0183531525220986,0.0984395027523984,
10.5081248887167));
#36420=CARTESIAN_POINT('Ctrl Pts',(0.0132379567575634,0.0992136050812441,
10.5116620905429));
#36421=CARTESIAN_POINT('Ctrl Pts',(0.00894444267269637,0.0995991814488194,
10.5141610714912));
#36422=CARTESIAN_POINT('Ctrl Pts',(0.0192962951151297,-0.10101340050352,
10.5309232968739));
#36423=CARTESIAN_POINT('Ctrl Pts',(0.0246829710160883,-0.100510889482336,
10.5276355936907));
#36424=CARTESIAN_POINT('Ctrl Pts',(0.0302700618807701,-0.0996151370866697,
10.5235433339832));
#36425=CARTESIAN_POINT('Ctrl Pts',(0.047446855001171,-0.095352727284558,
10.5101326862265));
#36426=CARTESIAN_POINT('Ctrl Pts',(0.0596224836125303,-0.0899496685517302,
10.4994713083419));
#36427=CARTESIAN_POINT('Ctrl Pts',(0.0803741273880472,-0.0743507192264208,
10.4812582586986));
#36428=CARTESIAN_POINT('Ctrl Pts',(0.0904178622326513,-0.0635857683883024,
10.4723242438985));
#36429=CARTESIAN_POINT('Ctrl Pts',(0.105408335734682,-0.0353360781276079,
10.4590400838768));
#36430=CARTESIAN_POINT('Ctrl Pts',(0.1146188438952,2.05947277554036E-14,
10.4509376050958));
#36431=CARTESIAN_POINT('Ctrl Pts',(0.10540833573468,0.035336078127622,10.4590400838768));
#36432=CARTESIAN_POINT('Ctrl Pts',(0.0904178622326502,0.0635857683883118,
10.4723242438985));
#36433=CARTESIAN_POINT('Ctrl Pts',(0.080374127388024,0.0743507192264434,
10.4812582586986));
#36434=CARTESIAN_POINT('Ctrl Pts',(0.0596224836125554,0.0899496685517165,
10.4994713083419));
#36435=CARTESIAN_POINT('Ctrl Pts',(0.0474468550011507,0.0953527272845648,
10.5101326862265));
#36436=CARTESIAN_POINT('Ctrl Pts',(0.0302700618807774,0.0996151370866677,
10.5235433339832));
#36437=CARTESIAN_POINT('Ctrl Pts',(0.0246829710160885,0.100510889482336,
10.5276355936907));
#36438=CARTESIAN_POINT('Ctrl Pts',(0.0192962951151303,0.10101340050352,
10.5309232968739));
#36439=CARTESIAN_POINT('Ctrl Pts',(0.0296481475575634,-0.102427619558221,
10.5476855222567));
#36440=CARTESIAN_POINT('Ctrl Pts',(0.0362443713099572,-0.101809611530983,
10.5435670582213));
#36441=CARTESIAN_POINT('Ctrl Pts',(0.0421748087255316,-0.100789286669114,
10.5389748496896));
#36442=CARTESIAN_POINT('Ctrl Pts',(0.0602984616063804,-0.0961969927156803,
10.524134695165));
#36443=CARTESIAN_POINT('Ctrl Pts',(0.0721769673050456,-0.0906177935398247,
10.5128816249181));
#36444=CARTESIAN_POINT('Ctrl Pts',(0.0922682177891075,-0.0747621107130237,
10.4934215201235));
#36445=CARTESIAN_POINT('Ctrl Pts',(0.101781264257295,-0.0638900076838062,
10.4838094232667));
#36446=CARTESIAN_POINT('Ctrl Pts',(0.115824116633652,-0.0354675295166492,
10.4694291815536));
#36447=CARTESIAN_POINT('Ctrl Pts',(0.124291726247609,8.66907190709113E-15,
10.4605209321096));
#36448=CARTESIAN_POINT('Ctrl Pts',(0.115824116633656,0.0354675295166414,
10.4694291815535));
#36449=CARTESIAN_POINT('Ctrl Pts',(0.101781264257307,0.06389000768379,10.4838094232667));
#36450=CARTESIAN_POINT('Ctrl Pts',(0.0922682177891217,0.0747621107130131,
10.4934215201235));
#36451=CARTESIAN_POINT('Ctrl Pts',(0.0721769673050495,0.0906177935398222,
10.5128816249181));
#36452=CARTESIAN_POINT('Ctrl Pts',(0.0602984616064044,0.0961969927156732,
10.524134695165));
#36453=CARTESIAN_POINT('Ctrl Pts',(0.0421748087255233,0.100789286669116,
10.5389748496896));
#36454=CARTESIAN_POINT('Ctrl Pts',(0.0362443713099577,0.101809611530983,
10.5435670582213));
#36455=CARTESIAN_POINT('Ctrl Pts',(0.0296481475575642,0.102427619558221,
10.5476855222567));
#36456=CARTESIAN_POINT('Ctrl Pts',(0.0399999999999971,-0.103841838612921,
10.5644477476394));
#36457=CARTESIAN_POINT('Ctrl Pts',(0.0476893855684823,-0.103106895932074,
10.5595405613692));
#36458=CARTESIAN_POINT('Ctrl Pts',(0.0540917180842104,-0.101964921003383,
10.5543932949561));
#36459=CARTESIAN_POINT('Ctrl Pts',(0.0730376207665544,-0.0970386918665594,
10.5381973744163));
#36460=CARTESIAN_POINT('Ctrl Pts',(0.0846768251420503,-0.0912869805493973,
10.5263171691939));
#36461=CARTESIAN_POINT('Ctrl Pts',(0.104130081685012,-0.0751729882392799,
10.5055930299794));
#36462=CARTESIAN_POINT('Ctrl Pts',(0.113106494285126,-0.0641959581874768,
10.4953286286927));
#36463=CARTESIAN_POINT('Ctrl Pts',(0.12619066965767,-0.0355990574058035,
10.4798181533174));
#36464=CARTESIAN_POINT('Ctrl Pts',(0.133920320923199,8.76610039849372E-15,
10.4701287368369));
#36465=CARTESIAN_POINT('Ctrl Pts',(0.126190669657674,0.0355990574057956,
10.4798181533174));
#36466=CARTESIAN_POINT('Ctrl Pts',(0.113106494285138,0.0641959581874607,
10.4953286286927));
#36467=CARTESIAN_POINT('Ctrl Pts',(0.104130081685026,0.0751729882392693,
10.5055930299794));
#36468=CARTESIAN_POINT('Ctrl Pts',(0.0846768251420541,0.0912869805493951,
10.5263171691939));
#36469=CARTESIAN_POINT('Ctrl Pts',(0.0730376207665783,0.0970386918665523,
10.5381973744163));
#36470=CARTESIAN_POINT('Ctrl Pts',(0.0540917180842021,0.101964921003385,
10.5543932949561));
#36471=CARTESIAN_POINT('Ctrl Pts',(0.0476893855684828,0.103106895932074,
10.5595405613692));
#36472=CARTESIAN_POINT('Ctrl Pts',(0.0399999999999982,0.103841838612921,
10.5644477476394));
#36473=CARTESIAN_POINT('',(0.0399999999999998,-0.103841838612921,10.5644477476394));
#36474=CARTESIAN_POINT('Ctrl Pts',(0.04,-0.103841838612921,10.5644477476394));
#36475=CARTESIAN_POINT('Ctrl Pts',(0.04,-0.102606877508547,10.5524412635046));
#36476=CARTESIAN_POINT('Ctrl Pts',(0.0399999999999991,-0.101164192447474,
10.5403304050204));
#36477=CARTESIAN_POINT('Ctrl Pts',(0.0399999999999991,-0.0972792884300837,
10.5159352723978));
#36478=CARTESIAN_POINT('Ctrl Pts',(0.0399999999999998,-0.0948285669211716,
10.5037338000625));
#36479=CARTESIAN_POINT('Ctrl Pts',(0.0399999999999998,-0.0916515138991173,
10.4916774593885));
#36480=CARTESIAN_POINT('',(0.0400000000000002,0.103841838612921,10.5644477476394));
#36481=CARTESIAN_POINT('Ctrl Pts',(0.0399999999999971,-0.103841838612921,
10.5644477476394));
#36482=CARTESIAN_POINT('Ctrl Pts',(0.0476893855684823,-0.103106895932074,
10.5595405613692));
#36483=CARTESIAN_POINT('Ctrl Pts',(0.0540917180842104,-0.101964921003383,
10.5543932949561));
#36484=CARTESIAN_POINT('Ctrl Pts',(0.0730376207665544,-0.0970386918665594,
10.5381973744163));
#36485=CARTESIAN_POINT('Ctrl Pts',(0.0846768251420503,-0.0912869805493973,
10.5263171691939));
#36486=CARTESIAN_POINT('Ctrl Pts',(0.104130081685012,-0.0751729882392799,
10.5055930299794));
#36487=CARTESIAN_POINT('Ctrl Pts',(0.113106494285126,-0.0641959581874768,
10.4953286286927));
#36488=CARTESIAN_POINT('Ctrl Pts',(0.12619066965767,-0.0355990574058035,
10.4798181533174));
#36489=CARTESIAN_POINT('Ctrl Pts',(0.133920320923199,8.76610039849372E-15,
10.4701287368369));
#36490=CARTESIAN_POINT('Ctrl Pts',(0.126190669657674,0.0355990574057956,
10.4798181533174));
#36491=CARTESIAN_POINT('Ctrl Pts',(0.113106494285138,0.0641959581874607,
10.4953286286927));
#36492=CARTESIAN_POINT('Ctrl Pts',(0.104130081685026,0.0751729882392693,
10.5055930299794));
#36493=CARTESIAN_POINT('Ctrl Pts',(0.0846768251420541,0.0912869805493951,
10.5263171691939));
#36494=CARTESIAN_POINT('Ctrl Pts',(0.0730376207665783,0.0970386918665523,
10.5381973744163));
#36495=CARTESIAN_POINT('Ctrl Pts',(0.0540917180842021,0.101964921003385,
10.5543932949561));
#36496=CARTESIAN_POINT('Ctrl Pts',(0.0476893855684828,0.103106895932074,
10.5595405613692));
#36497=CARTESIAN_POINT('Ctrl Pts',(0.0399999999999982,0.103841838612921,
10.5644477476394));
#36498=CARTESIAN_POINT('Ctrl Pts',(0.04,0.0916515138991168,10.4916774593885));
#36499=CARTESIAN_POINT('Ctrl Pts',(0.04,0.0935744633639231,10.4989747042521));
#36500=CARTESIAN_POINT('Ctrl Pts',(0.0399999999895264,0.095234686169019,
10.5063427163767));
#36501=CARTESIAN_POINT('Ctrl Pts',(0.0399999999895264,0.0999665537033885,
10.5306029708398));
#36502=CARTESIAN_POINT('Ctrl Pts',(0.0399999999999997,0.102095101447083,
10.5474656969538));
#36503=CARTESIAN_POINT('Ctrl Pts',(0.0399999999999997,0.103841838612921,
10.5644477476394));
#36504=CARTESIAN_POINT('Origin',(0.4,0.,10.45));
#36505=CARTESIAN_POINT('',(0.38,4.65365783675994E-17,10.45));
#36506=CARTESIAN_POINT('Origin',(0.,0.,10.45));
#36507=CARTESIAN_POINT('Ctrl Pts',(0.377017787534816,0.133632286077702,
10.58));
#36508=CARTESIAN_POINT('Ctrl Pts',(0.377017787534816,0.133632286077702,
10.5628264326263));
#36509=CARTESIAN_POINT('Ctrl Pts',(0.378257950025364,0.130263180113984,
10.5445759528919));
#36510=CARTESIAN_POINT('Ctrl Pts',(0.382671361121133,0.116705198842861,
10.5112796752359));
#36511=CARTESIAN_POINT('Ctrl Pts',(0.385743385887353,0.106539573413826,
10.4962244912617));
#36512=CARTESIAN_POINT('Ctrl Pts',(0.391476660649127,0.0830605783691531,
10.4724755856568));
#36513=CARTESIAN_POINT('Ctrl Pts',(0.39450689508103,0.068151397938132,10.4621678753065));
#36514=CARTESIAN_POINT('Ctrl Pts',(0.39881767731416,0.0351337186655312,
10.4484079854916));
#36515=CARTESIAN_POINT('Ctrl Pts',(0.400013024202683,0.0170314150408282,
10.4449835136144));
#36516=CARTESIAN_POINT('Ctrl Pts',(0.400012819411827,-0.0170559807859546,
10.4449833066593));
#36517=CARTESIAN_POINT('Ctrl Pts',(0.398817117536753,-0.0351583934957051,
10.4484074138439));
#36518=CARTESIAN_POINT('Ctrl Pts',(0.394505922058271,-0.0681763245922,10.4621668950494));
#36519=CARTESIAN_POINT('Ctrl Pts',(0.391475324666216,-0.0830858365898015,
10.4724741911262));
#36520=CARTESIAN_POINT('Ctrl Pts',(0.385741628020441,-0.106565333574474,
10.4962227929474));
#36521=CARTESIAN_POINT('Ctrl Pts',(0.382669212588462,-0.11673154779195,
10.5112770534905));
#36522=CARTESIAN_POINT('Ctrl Pts',(0.378255397171514,-0.130290214216898,
10.5445743531652));
#36523=CARTESIAN_POINT('Ctrl Pts',(0.377014663925107,-0.133660501471551,
10.5628181917482));
#36524=CARTESIAN_POINT('Ctrl Pts',(0.377014663925106,-0.133660501471554,
10.5971818082517));
#36525=CARTESIAN_POINT('Ctrl Pts',(0.378255397171518,-0.13029021421689,
10.6154256468348));
#36526=CARTESIAN_POINT('Ctrl Pts',(0.382669212588457,-0.116731547791971,
10.6487229465094));
#36527=CARTESIAN_POINT('Ctrl Pts',(0.385741628020435,-0.1065653335745,10.6637772070525));
#36528=CARTESIAN_POINT('Ctrl Pts',(0.39147532466622,-0.0830858365897902,
10.6875258088738));
#36529=CARTESIAN_POINT('Ctrl Pts',(0.394505922058272,-0.0681763245922005,
10.6978331049505));
#36530=CARTESIAN_POINT('Ctrl Pts',(0.398817117536754,-0.0351583934957121,
10.7115925861561));
#36531=CARTESIAN_POINT('Ctrl Pts',(0.400012819411829,-0.0170559807859655,
10.7150166933406));
#36532=CARTESIAN_POINT('Ctrl Pts',(0.400013024202684,0.0170314150408249,
10.7150164863856));
#36533=CARTESIAN_POINT('Ctrl Pts',(0.398817677314164,0.0351337186655008,
10.7115920145084));
#36534=CARTESIAN_POINT('Ctrl Pts',(0.394506895081026,0.068151397938163,
10.6978321246935));
#36535=CARTESIAN_POINT('Ctrl Pts',(0.391476660649127,0.0830605783691558,
10.6875244143432));
#36536=CARTESIAN_POINT('Ctrl Pts',(0.385743385887349,0.106539573413844,
10.6637755087383));
#36537=CARTESIAN_POINT('Ctrl Pts',(0.382671361121131,0.116705198842871,
10.6487203247641));
#36538=CARTESIAN_POINT('Ctrl Pts',(0.378257950025365,0.130263180113984,
10.6154240471081));
#36539=CARTESIAN_POINT('Ctrl Pts',(0.377017787534816,0.133632286077702,
10.5971735673738));
#36540=CARTESIAN_POINT('Ctrl Pts',(0.377017787534816,0.133632286077702,
10.58));
#36541=CARTESIAN_POINT('Ctrl Pts',(0.370002790679512,0.124088190718468,
10.58));
#36542=CARTESIAN_POINT('Ctrl Pts',(0.370006405685752,0.124088635524633,
10.5637880731882));
#36543=CARTESIAN_POINT('Ctrl Pts',(0.371101921434292,0.120800521232035,
10.5465693309555));
#36544=CARTESIAN_POINT('Ctrl Pts',(0.374989826903314,0.107735332893418,
10.5153991323168));
#36545=CARTESIAN_POINT('Ctrl Pts',(0.377685178239063,0.0980280855761085,
10.5014498597172));
#36546=CARTESIAN_POINT('Ctrl Pts',(0.382674879286364,0.0759567643144633,
10.4796760923536));
#36547=CARTESIAN_POINT('Ctrl Pts',(0.385295227322924,0.062110380135337,
10.4703530240385));
#36548=CARTESIAN_POINT('Ctrl Pts',(0.388992255115961,0.0318559581336749,
10.4580194294971));
#36549=CARTESIAN_POINT('Ctrl Pts',(0.390011657552353,0.0154317369722092,
10.4549861845637));
#36550=CARTESIAN_POINT('Ctrl Pts',(0.390011508655186,-0.0154563035124759,
10.4549859776087));
#36551=CARTESIAN_POINT('Ctrl Pts',(0.388991613942717,-0.0318806292414934,
10.4580188578494));
#36552=CARTESIAN_POINT('Ctrl Pts',(0.3852943745433,-0.0621353133809165,
10.4703520437814));
#36553=CARTESIAN_POINT('Ctrl Pts',(0.3826733055481,-0.0759820082990766,
10.479674697823));
#36554=CARTESIAN_POINT('Ctrl Pts',(0.37768379836919,-0.0980538687874221,
10.5014481614029));
#36555=CARTESIAN_POINT('Ctrl Pts',(0.374986900891037,-0.107761633235289,
10.5153965105715));
#36556=CARTESIAN_POINT('Ctrl Pts',(0.371100617680385,-0.120827636867808,
10.5465677312288));
#36557=CARTESIAN_POINT('Ctrl Pts',(0.370000627774456,-0.124116615118387,
10.5637798323102));
#36558=CARTESIAN_POINT('Ctrl Pts',(0.370000627774456,-0.12411661511839,
10.5962201676897));
#36559=CARTESIAN_POINT('Ctrl Pts',(0.371100617680389,-0.1208276368678,10.6134322687712));
#36560=CARTESIAN_POINT('Ctrl Pts',(0.374986900891032,-0.10776163323531,
10.6446034894284));
#36561=CARTESIAN_POINT('Ctrl Pts',(0.377683798369184,-0.098053868787448,
10.658551838597));
#36562=CARTESIAN_POINT('Ctrl Pts',(0.382673305548104,-0.0759820082990655,
10.680325302177));
#36563=CARTESIAN_POINT('Ctrl Pts',(0.385294374543301,-0.062135313380917,
10.6896479562185));
#36564=CARTESIAN_POINT('Ctrl Pts',(0.388991613942718,-0.0318806292415004,
10.7019811421505));
#36565=CARTESIAN_POINT('Ctrl Pts',(0.390011508655187,-0.0154563035124868,
10.7050140223912));
#36566=CARTESIAN_POINT('Ctrl Pts',(0.390011657552354,0.0154317369722058,
10.7050138154362));
#36567=CARTESIAN_POINT('Ctrl Pts',(0.388992255115965,0.0318559581336445,
10.7019805705029));
#36568=CARTESIAN_POINT('Ctrl Pts',(0.38529522732292,0.0621103801353678,
10.6896469759614));
#36569=CARTESIAN_POINT('Ctrl Pts',(0.382674879286364,0.075956764314466,
10.6803239076464));
#36570=CARTESIAN_POINT('Ctrl Pts',(0.377685178239059,0.0980280855761259,
10.6585501402828));
#36571=CARTESIAN_POINT('Ctrl Pts',(0.374989826903312,0.107735332893429,
10.6446008676831));
#36572=CARTESIAN_POINT('Ctrl Pts',(0.371101921434293,0.120800521232036,
10.6134306690445));
#36573=CARTESIAN_POINT('Ctrl Pts',(0.370006405685752,0.124088635524634,
10.5962119268118));
#36574=CARTESIAN_POINT('Ctrl Pts',(0.370002790679512,0.124088190718468,
10.58));
#36575=CARTESIAN_POINT('Ctrl Pts',(0.362987793824209,0.114544095359234,
10.58));
#36576=CARTESIAN_POINT('Ctrl Pts',(0.362984178817969,0.114543650553069,
10.5647559738531));
#36577=CARTESIAN_POINT('Ctrl Pts',(0.363944180231836,0.111328542612427,
10.548562151861));
#36578=CARTESIAN_POINT('Ctrl Pts',(0.367306317957412,0.0987741164193237,
10.5195209482943));
#36579=CARTESIAN_POINT('Ctrl Pts',(0.369622188878733,0.0895126083068797,
10.5066817992144));
#36580=CARTESIAN_POINT('Ctrl Pts',(0.373874212172674,0.0688567722200343,
10.4868715827257));
#36581=CARTESIAN_POINT('Ctrl Pts',(0.376076337898789,0.0560754474460455,
10.4785490202942));
#36582=CARTESIAN_POINT('Ctrl Pts',(0.37917104833718,0.0285718270842341,
10.4676207455255));
#36583=CARTESIAN_POINT('Ctrl Pts',(0.380009038186307,0.013843656528979,
10.4649889870543));
#36584=CARTESIAN_POINT('Ctrl Pts',(0.380008842010176,-0.0138687919798646,
10.4649887173818));
#36585=CARTESIAN_POINT('Ctrl Pts',(0.37917074628356,-0.0285970786710002,
10.4676200006407));
#36586=CARTESIAN_POINT('Ctrl Pts',(0.376075551131707,-0.0561009463910287,
10.4785477429714));
#36587=CARTESIAN_POINT('Ctrl Pts',(0.37387353477512,-0.0688826312592696,
10.4868697655843));
#36588=CARTESIAN_POINT('Ctrl Pts',(0.369620606736793,-0.0895389436561773,
10.506679586228));
#36589=CARTESIAN_POINT('Ctrl Pts',(0.367305623684723,-0.0988011258886412,
10.5195175320322));
#36590=CARTESIAN_POINT('Ctrl Pts',(0.363941182418194,-0.111356123007109,
10.5485600673391));
#36591=CARTESIAN_POINT('Ctrl Pts',(0.362984693436124,-0.114572757005271,
10.5647452355871));
#36592=CARTESIAN_POINT('Ctrl Pts',(0.362984693436123,-0.114572757005271,
10.5952547644128));
#36593=CARTESIAN_POINT('Ctrl Pts',(0.363941182418194,-0.111356123007106,
10.6114399326608));
#36594=CARTESIAN_POINT('Ctrl Pts',(0.367305623684722,-0.0988011258886432,
10.6404824679677));
#36595=CARTESIAN_POINT('Ctrl Pts',(0.369620606736792,-0.0895389436561786,
10.6533204137719));
#36596=CARTESIAN_POINT('Ctrl Pts',(0.37387353477512,-0.0688826312592703,
10.6731302344156));
#36597=CARTESIAN_POINT('Ctrl Pts',(0.376075551131706,-0.0561009463910289,
10.6814522570286));
#36598=CARTESIAN_POINT('Ctrl Pts',(0.37917074628356,-0.028597078670995,
10.6923799993593));
#36599=CARTESIAN_POINT('Ctrl Pts',(0.380008842010175,-0.0138687919798612,
10.6950112826181));
#36600=CARTESIAN_POINT('Ctrl Pts',(0.380009038186307,0.0138436565289819,
10.6950110129456));
#36601=CARTESIAN_POINT('Ctrl Pts',(0.379171048337179,0.0285718270842431,
10.6923792544745));
#36602=CARTESIAN_POINT('Ctrl Pts',(0.37607633789879,0.0560754474460394,
10.6814509797058));
#36603=CARTESIAN_POINT('Ctrl Pts',(0.373874212172674,0.0688567722200364,
10.6731284172743));
#36604=CARTESIAN_POINT('Ctrl Pts',(0.369622188878734,0.0895126083068803,
10.6533182007855));
#36605=CARTESIAN_POINT('Ctrl Pts',(0.367306317957412,0.0987741164193243,
10.6404790517057));
#36606=CARTESIAN_POINT('Ctrl Pts',(0.363944180231836,0.111328542612426,
10.611437848139));
#36607=CARTESIAN_POINT('Ctrl Pts',(0.362984178817969,0.114543650553068,
10.5952440261469));
#36608=CARTESIAN_POINT('Ctrl Pts',(0.362987793824209,0.114544095359234,
10.58));
#36609=CARTESIAN_POINT('Ctrl Pts',(0.355972796968906,0.105,10.58));
#36610=CARTESIAN_POINT('Ctrl Pts',(0.355972796968906,0.105,10.5657176144151));
#36611=CARTESIAN_POINT('Ctrl Pts',(0.356788151640763,0.101865883730478,
10.5505555299246));
#36612=CARTESIAN_POINT('Ctrl Pts',(0.359624783739593,0.0898042504698815,
10.5236404053753));
#36613=CARTESIAN_POINT('Ctrl Pts',(0.361563981230443,0.0810011204691618,
10.5119071676699));
#36614=CARTESIAN_POINT('Ctrl Pts',(0.365072430809911,0.0617529581653445,
10.4940720894225));
#36615=CARTESIAN_POINT('Ctrl Pts',(0.366864670140683,0.0500344296432505,
10.4867341690262));
#36616=CARTESIAN_POINT('Ctrl Pts',(0.369345626138981,0.0252940665523777,
10.477232189531));
#36617=CARTESIAN_POINT('Ctrl Pts',(0.370007671535977,0.01224397846036,10.4749916580037));
#36618=CARTESIAN_POINT('Ctrl Pts',(0.370007531253534,-0.0122691147063859,
10.4749913883312));
#36619=CARTESIAN_POINT('Ctrl Pts',(0.369345242689524,-0.0253193144167885,
10.4772314446462));
#36620=CARTESIAN_POINT('Ctrl Pts',(0.366864003616736,-0.0500599351797451,
10.4867328917034));
#36621=CARTESIAN_POINT('Ctrl Pts',(0.365071515657005,-0.0617788029685447,
10.4940702722811));
#36622=CARTESIAN_POINT('Ctrl Pts',(0.361562777085542,-0.0810274788691257,
10.5119049546835));
#36623=CARTESIAN_POINT('Ctrl Pts',(0.359623311987298,-0.0898312113319797,
10.5236369891132));
#36624=CARTESIAN_POINT('Ctrl Pts',(0.356786402927065,-0.101893545658019,
10.5505534454027));
#36625=CARTESIAN_POINT('Ctrl Pts',(0.355970657285474,-0.105028870652107,
10.5657068761491));
#36626=CARTESIAN_POINT('Ctrl Pts',(0.355970657285473,-0.105028870652107,
10.5942931238509));
#36627=CARTESIAN_POINT('Ctrl Pts',(0.356786402927066,-0.101893545658015,
10.6094465545972));
#36628=CARTESIAN_POINT('Ctrl Pts',(0.359623311987297,-0.0898312113319818,
10.6363630108867));
#36629=CARTESIAN_POINT('Ctrl Pts',(0.361562777085541,-0.0810274788691267,
10.6480950453164));
#36630=CARTESIAN_POINT('Ctrl Pts',(0.365071515657004,-0.0617788029685456,
10.6659297277188));
#36631=CARTESIAN_POINT('Ctrl Pts',(0.366864003616735,-0.0500599351797454,
10.6732671082965));
#36632=CARTESIAN_POINT('Ctrl Pts',(0.369345242689524,-0.0253193144167833,
10.6827685553537));
#36633=CARTESIAN_POINT('Ctrl Pts',(0.370007531253534,-0.0122691147063825,
10.6850086116688));
#36634=CARTESIAN_POINT('Ctrl Pts',(0.370007671535977,0.0122439784603628,
10.6850083419962));
#36635=CARTESIAN_POINT('Ctrl Pts',(0.36934562613898,0.0252940665523868,
10.6827678104689));
#36636=CARTESIAN_POINT('Ctrl Pts',(0.366864670140684,0.0500344296432442,
10.6732658309738));
#36637=CARTESIAN_POINT('Ctrl Pts',(0.365072430809911,0.0617529581653465,
10.6659279105774));
#36638=CARTESIAN_POINT('Ctrl Pts',(0.361563981230444,0.0810011204691621,
10.6480928323301));
#36639=CARTESIAN_POINT('Ctrl Pts',(0.359624783739593,0.0898042504698822,
10.6363595946247));
#36640=CARTESIAN_POINT('Ctrl Pts',(0.356788151640764,0.101865883730477,
10.6094444700754));
#36641=CARTESIAN_POINT('Ctrl Pts',(0.355972796968906,0.105,10.5942823855849));
#36642=CARTESIAN_POINT('Ctrl Pts',(0.355972796968906,0.105,10.58));
#36643=CARTESIAN_POINT('',(0.392324587256711,-0.0779994227069357,10.4700129327839));
#36644=CARTESIAN_POINT('',(0.38750984162879,-1.13350214458844E-5,10.4574879118198));
#36645=CARTESIAN_POINT('Ctrl Pts',(0.392324587256711,-0.0779994227069357,
10.4700129327839));
#36646=CARTESIAN_POINT('Ctrl Pts',(0.3914179472595,-0.0710898798500254,
10.4677824164029));
#36647=CARTESIAN_POINT('Ctrl Pts',(0.390647674347867,-0.0640945112802287,
10.4658141254007));
#36648=CARTESIAN_POINT('Ctrl Pts',(0.390006979063182,-0.057004463951378,
10.4641394037107));
#36649=CARTESIAN_POINT('Ctrl Pts',(0.389738309424129,-0.0540313182107284,
10.4634371246668));
#36650=CARTESIAN_POINT('Ctrl Pts',(0.389492752976518,-0.0510460578652142,
10.4627882375969));
#36651=CARTESIAN_POINT('Ctrl Pts',(0.389268637081754,-0.0480486678529736,
10.4621981307677));
#36652=CARTESIAN_POINT('Ctrl Pts',(0.388773697289598,-0.0414292016556794,
10.4608949329213));
#36653=CARTESIAN_POINT('Ctrl Pts',(0.388374227255805,-0.0347520280387355,
10.4598756996778));
#36654=CARTESIAN_POINT('Ctrl Pts',(0.388086077313271,-0.0280389018830262,
10.4591141553202));
#36655=CARTESIAN_POINT('Ctrl Pts',(0.387922086290066,-0.0242183478426609,
10.4586807475003));
#36656=CARTESIAN_POINT('Ctrl Pts',(0.387793898518198,-0.0203854294882888,
10.4583313532265));
#36657=CARTESIAN_POINT('Ctrl Pts',(0.38770134624721,-0.016541244006537,
10.458067528716));
#36658=CARTESIAN_POINT('Ctrl Pts',(0.387628168683527,-0.0135017926252255,
10.4578589327009));
#36659=CARTESIAN_POINT('Ctrl Pts',(0.387577297833347,-0.0104585822931131,
10.4577041418123));
#36660=CARTESIAN_POINT('Ctrl Pts',(0.387546792306271,-0.00741190850063314,
10.457606743657));
#36661=CARTESIAN_POINT('Ctrl Pts',(0.387530351373301,-0.00576990574219154,
10.4575542509877));
#36662=CARTESIAN_POINT('Ctrl Pts',(0.387519801015628,-0.00412720254292159,
10.4575184923917));
#36663=CARTESIAN_POINT('Ctrl Pts',(0.387514611538262,-0.00248401466470584,
10.4575004335314));
#36664=CARTESIAN_POINT('Ctrl Pts',(0.387512010291039,-0.00166035987157767,
10.4574913814522));
#36665=CARTESIAN_POINT('Ctrl Pts',(0.387510753131607,-0.000834836263530225,
10.4574867801339));
#36666=CARTESIAN_POINT('Ctrl Pts',(0.387510757804169,-1.23902195018747E-5,
10.4574867865088));
#36667=CARTESIAN_POINT('',(0.392324929054758,0.0779792774862667,10.4700112775181));
#36668=CARTESIAN_POINT('Ctrl Pts',(0.387510757804169,-1.23902195018771E-5,
10.4574867865088));
#36669=CARTESIAN_POINT('Ctrl Pts',(0.387510760917883,0.000525053166309368,
10.4574867906143));
#36670=CARTESIAN_POINT('Ctrl Pts',(0.387511301666096,0.00106361088239916,
10.4574887586056));
#36671=CARTESIAN_POINT('Ctrl Pts',(0.387512404993374,0.00160185431838427,
10.4574926511551));
#36672=CARTESIAN_POINT('Ctrl Pts',(0.38751555332776,0.00313772708404272,
10.4575037585098));
#36673=CARTESIAN_POINT('Ctrl Pts',(0.387523288659664,0.00467326443951501,
10.4575305065774));
#36674=CARTESIAN_POINT('Ctrl Pts',(0.387536072247131,0.00620825863535256,
10.4575720543493));
#36675=CARTESIAN_POINT('Ctrl Pts',(0.387557367005732,0.00876523498789927,
10.4576412641682));
#36676=CARTESIAN_POINT('Ctrl Pts',(0.387592709089323,0.0113200607878381,
10.4577514381998));
#36677=CARTESIAN_POINT('Ctrl Pts',(0.387643462116037,0.013872445644174,
10.4579000655362));
#36678=CARTESIAN_POINT('Ctrl Pts',(0.387745259086891,0.0189918456809811,
10.4581981721439));
#36679=CARTESIAN_POINT('Ctrl Pts',(0.387909563732894,0.0240968961657213,
10.4586494962418));
#36680=CARTESIAN_POINT('Ctrl Pts',(0.388138027023152,0.0291870207304549,
10.4592504297026));
#36681=CARTESIAN_POINT('Ctrl Pts',(0.38842171987062,0.0355076507542359,
10.4599966350314));
#36682=CARTESIAN_POINT('Ctrl Pts',(0.388803515452204,0.041793505019326,
10.460972224136));
#36683=CARTESIAN_POINT('Ctrl Pts',(0.389269380504044,0.0480237819441658,
10.4621989247368));
#36684=CARTESIAN_POINT('Ctrl Pts',(0.389445324894814,0.0503767858313245,
10.4626622157456));
#36685=CARTESIAN_POINT('Ctrl Pts',(0.389634435791483,0.0527216898232129,
10.4631616413639));
#36686=CARTESIAN_POINT('Ctrl Pts',(0.389837537339329,0.0550584657624432,
10.4636944184715));
#36687=CARTESIAN_POINT('Ctrl Pts',(0.390433239144012,0.0619122867150533,
10.4652570667517));
#36688=CARTESIAN_POINT('Ctrl Pts',(0.391148398175305,0.0686769039822018,
10.4670981722794));
#36689=CARTESIAN_POINT('Ctrl Pts',(0.391990110278716,0.0753629866058349,
10.4691851390505));
#36690=CARTESIAN_POINT('Ctrl Pts',(0.392099863338824,0.0762348025451608,
10.4694572641495));
#36691=CARTESIAN_POINT('Ctrl Pts',(0.392211757415364,0.077105234082072,
10.4697336199639));
#36692=CARTESIAN_POINT('Ctrl Pts',(0.392325801285573,0.0779742601298161,
10.4700141742871));
#36693=CARTESIAN_POINT('',(0.377017787534816,0.133632286077702,10.58));
#36694=CARTESIAN_POINT('Ctrl Pts',(0.392325801275538,0.0779742601803755,
10.4700141743233));
#36695=CARTESIAN_POINT('Ctrl Pts',(0.391112328098889,0.0840879572291327,
10.4744019432579));
#36696=CARTESIAN_POINT('Ctrl Pts',(0.389846070963454,0.0897381943461625,
10.4792299663789));
#36697=CARTESIAN_POINT('Ctrl Pts',(0.385743385887353,0.106539573413826,
10.4962244912617));
#36698=CARTESIAN_POINT('Ctrl Pts',(0.382671361121133,0.116705198842861,
10.5112796752359));
#36699=CARTESIAN_POINT('Ctrl Pts',(0.378257950025364,0.130263180113984,
10.5445759528919));
#36700=CARTESIAN_POINT('Ctrl Pts',(0.377017787534816,0.133632286077702,
10.5628264326263));
#36701=CARTESIAN_POINT('Ctrl Pts',(0.377017787534816,0.133632286077702,
10.58));
#36702=CARTESIAN_POINT('',(0.355972796968906,0.105,10.58));
#36703=CARTESIAN_POINT('',(0.377017787534816,0.133632286077702,10.58));
#36704=CARTESIAN_POINT('',(0.355970657285473,-0.105028870652107,10.58));
#36705=CARTESIAN_POINT('Ctrl Pts',(0.355972796968906,0.105,10.58));
#36706=CARTESIAN_POINT('Ctrl Pts',(0.355972796968906,0.105,10.5657176144151));
#36707=CARTESIAN_POINT('Ctrl Pts',(0.356788151640763,0.101865883730478,
10.5505555299246));
#36708=CARTESIAN_POINT('Ctrl Pts',(0.359624783739593,0.0898042504698815,
10.5236404053753));
#36709=CARTESIAN_POINT('Ctrl Pts',(0.361563981230443,0.0810011204691618,
10.5119071676699));
#36710=CARTESIAN_POINT('Ctrl Pts',(0.365072430809911,0.0617529581653445,
10.4940720894225));
#36711=CARTESIAN_POINT('Ctrl Pts',(0.366864670140683,0.0500344296432505,
10.4867341690262));
#36712=CARTESIAN_POINT('Ctrl Pts',(0.369345626138981,0.0252940665523777,
10.477232189531));
#36713=CARTESIAN_POINT('Ctrl Pts',(0.370007671535977,0.01224397846036,10.4749916580037));
#36714=CARTESIAN_POINT('Ctrl Pts',(0.370007531253534,-0.0122691147063859,
10.4749913883312));
#36715=CARTESIAN_POINT('Ctrl Pts',(0.369345242689524,-0.0253193144167885,
10.4772314446462));
#36716=CARTESIAN_POINT('Ctrl Pts',(0.366864003616736,-0.0500599351797451,
10.4867328917034));
#36717=CARTESIAN_POINT('Ctrl Pts',(0.365071515657005,-0.0617788029685447,
10.4940702722811));
#36718=CARTESIAN_POINT('Ctrl Pts',(0.361562777085542,-0.0810274788691257,
10.5119049546835));
#36719=CARTESIAN_POINT('Ctrl Pts',(0.359623311987298,-0.0898312113319797,
10.5236369891132));
#36720=CARTESIAN_POINT('Ctrl Pts',(0.356786402927065,-0.101893545658019,
10.5505534454027));
#36721=CARTESIAN_POINT('Ctrl Pts',(0.355970657285474,-0.105028870652107,
10.5657068761491));
#36722=CARTESIAN_POINT('Ctrl Pts',(0.355970657285473,-0.105028870652107,
10.58));
#36723=CARTESIAN_POINT('Ctrl Pts',(0.355970657285473,-0.105028870652107,
10.58));
#36724=CARTESIAN_POINT('Ctrl Pts',(0.355970657285473,-0.105028870652107,
10.5942931238509));
#36725=CARTESIAN_POINT('Ctrl Pts',(0.356786402927066,-0.101893545658015,
10.6094465545972));
#36726=CARTESIAN_POINT('Ctrl Pts',(0.359623311987297,-0.0898312113319818,
10.6363630108867));
#36727=CARTESIAN_POINT('Ctrl Pts',(0.361562777085541,-0.0810274788691267,
10.6480950453164));
#36728=CARTESIAN_POINT('Ctrl Pts',(0.365071515657004,-0.0617788029685456,
10.6659297277188));
#36729=CARTESIAN_POINT('Ctrl Pts',(0.366864003616735,-0.0500599351797454,
10.6732671082965));
#36730=CARTESIAN_POINT('Ctrl Pts',(0.369345242689524,-0.0253193144167833,
10.6827685553537));
#36731=CARTESIAN_POINT('Ctrl Pts',(0.370007531253534,-0.0122691147063825,
10.6850086116688));
#36732=CARTESIAN_POINT('Ctrl Pts',(0.370007671535977,0.0122439784603628,
10.6850083419962));
#36733=CARTESIAN_POINT('Ctrl Pts',(0.36934562613898,0.0252940665523868,
10.6827678104689));
#36734=CARTESIAN_POINT('Ctrl Pts',(0.366864670140684,0.0500344296432442,
10.6732658309738));
#36735=CARTESIAN_POINT('Ctrl Pts',(0.365072430809911,0.0617529581653465,
10.6659279105774));
#36736=CARTESIAN_POINT('Ctrl Pts',(0.361563981230444,0.0810011204691621,
10.6480928323301));
#36737=CARTESIAN_POINT('Ctrl Pts',(0.359624783739593,0.0898042504698822,
10.6363595946247));
#36738=CARTESIAN_POINT('Ctrl Pts',(0.356788151640764,0.101865883730477,
10.6094444700754));
#36739=CARTESIAN_POINT('Ctrl Pts',(0.355972796968906,0.105,10.5942823855849));
#36740=CARTESIAN_POINT('Ctrl Pts',(0.355972796968906,0.105,10.58));
#36741=CARTESIAN_POINT('',(0.398342724806441,0.0363740785969918,10.7099999999999));
#36742=CARTESIAN_POINT('Ctrl Pts',(0.377017787534816,0.133632286077702,
10.58));
#36743=CARTESIAN_POINT('Ctrl Pts',(0.377017787534816,0.133632286077702,
10.5971735673738));
#36744=CARTESIAN_POINT('Ctrl Pts',(0.378257950025365,0.130263180113984,
10.6154240471081));
#36745=CARTESIAN_POINT('Ctrl Pts',(0.382671361121131,0.116705198842871,
10.6487203247641));
#36746=CARTESIAN_POINT('Ctrl Pts',(0.385743385887349,0.106539573413844,
10.6637755087383));
#36747=CARTESIAN_POINT('Ctrl Pts',(0.391476660649127,0.0830605783691558,
10.6875244143432));
#36748=CARTESIAN_POINT('Ctrl Pts',(0.394506895081026,0.068151397938163,
10.6978321246935));
#36749=CARTESIAN_POINT('Ctrl Pts',(0.397311776340776,0.0466679026410903,
10.7067852229923));
#36750=CARTESIAN_POINT('Ctrl Pts',(0.397874093042254,0.0415485580836963,
10.7085446143007));
#36751=CARTESIAN_POINT('Ctrl Pts',(0.398342795273631,0.0363570891554297,
10.7099910945945));
#36752=CARTESIAN_POINT('',(0.398342724806499,-0.03637407859636,10.71));
#36753=CARTESIAN_POINT('Ctrl Pts',(0.398342247906153,-0.0363817831807788,
10.7099916508698));
#36754=CARTESIAN_POINT('Ctrl Pts',(0.397665066396712,-0.0326461425599149,
10.7099853342879));
#36755=CARTESIAN_POINT('Ctrl Pts',(0.397083002923767,-0.0288995863484758,
10.7099810242112));
#36756=CARTESIAN_POINT('Ctrl Pts',(0.396604742785928,-0.0251364196314169,
10.7099811705733));
#36757=CARTESIAN_POINT('Ctrl Pts',(0.395872802041393,-0.0193771793544803,
10.7099813945695));
#36758=CARTESIAN_POINT('Ctrl Pts',(0.395389651144243,-0.0136148183112041,
10.7099940233747));
#36759=CARTESIAN_POINT('Ctrl Pts',(0.395163312234515,-0.00781210949747046,
10.7100055875414));
#36760=CARTESIAN_POINT('Ctrl Pts',(0.39510698933434,-0.00636814482673823,
10.7100084652058));
#36761=CARTESIAN_POINT('Ctrl Pts',(0.395066553089786,-0.00492380828909155,
10.7100110998838));
#36762=CARTESIAN_POINT('Ctrl Pts',(0.395041766952865,-0.00347852169201901,
10.7100129042549));
#36763=CARTESIAN_POINT('Ctrl Pts',(0.39502804355889,-0.00267830673951237,
10.710013903285));
#36764=CARTESIAN_POINT('Ctrl Pts',(0.395019119897156,-0.00187802612202232,
10.7100146444282));
#36765=CARTESIAN_POINT('Ctrl Pts',(0.395014934638734,-0.00107759250488598,
10.7100150047607));
#36766=CARTESIAN_POINT('Ctrl Pts',(0.39501307801116,-0.00072251117550288,
10.7100151646083));
#36767=CARTESIAN_POINT('Ctrl Pts',(0.395012153921115,-0.000367158428743391,
10.7100152493742));
#36768=CARTESIAN_POINT('Ctrl Pts',(0.395012155839313,-1.23041126689258E-5,
10.7100152469662));
#36769=CARTESIAN_POINT('Ctrl Pts',(0.39501215756284,0.000306537193240153,
10.7100152448027));
#36770=CARTESIAN_POINT('Ctrl Pts',(0.39501290706911,0.000625760855678687,
10.71001517254));
#36771=CARTESIAN_POINT('Ctrl Pts',(0.395014408943175,0.000944808589093608,
10.7100150384837));
#36772=CARTESIAN_POINT('Ctrl Pts',(0.395018110328239,0.00173110521886498,
10.7100147081003));
#36773=CARTESIAN_POINT('Ctrl Pts',(0.395026381611087,0.00251725892388332,
10.7100140041378));
#36774=CARTESIAN_POINT('Ctrl Pts',(0.395039281660777,0.00330335200016204,
10.7100130440316));
#36775=CARTESIAN_POINT('Ctrl Pts',(0.395061946304566,0.0046844722273079,
10.7100113571803));
#36776=CARTESIAN_POINT('Ctrl Pts',(0.395098893168343,0.00606475624817226,
10.7100088886225));
#36777=CARTESIAN_POINT('Ctrl Pts',(0.395150336257454,0.00744470557640811,
10.7100061596766));
#36778=CARTESIAN_POINT('Ctrl Pts',(0.395255859270476,0.0102753367350618,
10.7100005619064));
#36779=CARTESIAN_POINT('Ctrl Pts',(0.395422268232612,0.0130994926770529,
10.7099940194268));
#36780=CARTESIAN_POINT('Ctrl Pts',(0.39564974640504,0.0159218010131768,
10.709989245592));
#36781=CARTESIAN_POINT('Ctrl Pts',(0.396153036495399,0.0221660916294672,
10.7099786835951));
#36782=CARTESIAN_POINT('Ctrl Pts',(0.396952990163372,0.028357002547276,
10.7099791005708));
#36783=CARTESIAN_POINT('Ctrl Pts',(0.398019360427533,0.0345300530562236,
10.7099882094322));
#36784=CARTESIAN_POINT('Ctrl Pts',(0.398124600500028,0.0351392713595705,
10.7099891083857));
#36785=CARTESIAN_POINT('Ctrl Pts',(0.3982324238991,0.035748280023644,10.7099900739033));
#36786=CARTESIAN_POINT('Ctrl Pts',(0.398342795273687,0.0363570891548118,
10.7099910945946));
#36787=CARTESIAN_POINT('Ctrl Pts',(0.398342247906152,-0.0363817831807865,
10.7099916508698));
#36788=CARTESIAN_POINT('Ctrl Pts',(0.397873464638273,-0.0415732844705318,
10.7085452525623));
#36789=CARTESIAN_POINT('Ctrl Pts',(0.397311072202917,-0.0466926654416248,
10.706785937381));
#36790=CARTESIAN_POINT('Ctrl Pts',(0.394505922058272,-0.0681763245922005,
10.6978331049505));
#36791=CARTESIAN_POINT('Ctrl Pts',(0.39147532466622,-0.0830858365897902,
10.6875258088738));
#36792=CARTESIAN_POINT('Ctrl Pts',(0.385741628020435,-0.1065653335745,10.6637772070525));
#36793=CARTESIAN_POINT('Ctrl Pts',(0.382669212588457,-0.116731547791971,
10.6487229465094));
#36794=CARTESIAN_POINT('Ctrl Pts',(0.378255397171518,-0.13029021421689,
10.6154256468348));
#36795=CARTESIAN_POINT('Ctrl Pts',(0.377014663925106,-0.133660501471554,
10.5971818082517));
#36796=CARTESIAN_POINT('Ctrl Pts',(0.377014663925107,-0.133660501471551,
10.5628181917482));
#36797=CARTESIAN_POINT('Ctrl Pts',(0.378255397171514,-0.130290214216898,
10.5445743531652));
#36798=CARTESIAN_POINT('Ctrl Pts',(0.382669212588462,-0.11673154779195,
10.5112770534905));
#36799=CARTESIAN_POINT('Ctrl Pts',(0.385741628020441,-0.106565333574474,
10.4962227929474));
#36800=CARTESIAN_POINT('Ctrl Pts',(0.389844614775671,-0.0897635962138861,
10.4792284863512));
#36801=CARTESIAN_POINT('Ctrl Pts',(0.391110990879574,-0.0841132370178976,
10.4744005782828));
#36802=CARTESIAN_POINT('Ctrl Pts',(0.392324586605502,-0.0779994259875773,
10.4700129351383));
#36803=CARTESIAN_POINT('Origin',(0.,0.,10.58));
#36804=CARTESIAN_POINT('Origin',(0.,0.,10.47));
#36805=CARTESIAN_POINT('Origin',(0.,0.,10.71));
#36806=CARTESIAN_POINT('Origin',(0.,0.,10.46));
#36807=CARTESIAN_POINT('',(0.39,4.77612251667468E-17,10.46));
#36808=CARTESIAN_POINT('Origin',(0.245,0.,10.58));
#36809=CARTESIAN_POINT('',(0.0400000000000001,0.103841838612921,10.5955522523606));
#36810=CARTESIAN_POINT('',(0.0400000000000005,-0.103841838612921,10.5955522523606));
#36811=CARTESIAN_POINT('Ctrl Pts',(0.0399999999999981,0.103841838612921,
10.5955522523606));
#36812=CARTESIAN_POINT('Ctrl Pts',(0.0476893855684824,0.103106895932074,
10.6004594386308));
#36813=CARTESIAN_POINT('Ctrl Pts',(0.0540917217987843,0.101964920739599,
10.6056067063421));
#36814=CARTESIAN_POINT('Ctrl Pts',(0.0730376318384075,0.0970386910483417,
10.6218026292622));
#36815=CARTESIAN_POINT('Ctrl Pts',(0.0846768485016188,0.0912869792271611,
10.6336828384074));
#36816=CARTESIAN_POINT('Ctrl Pts',(0.10413011273211,0.0751729867880902,
10.6544069799274));
#36817=CARTESIAN_POINT('Ctrl Pts',(0.113106530347439,0.0641959568676023,
10.6646713825649));
#36818=CARTESIAN_POINT('Ctrl Pts',(0.12619070930351,0.0355990566133719,
10.6801818582265));
#36819=CARTESIAN_POINT('Ctrl Pts',(0.13392036430385,-1.94332703229122E-14,
10.6898712751113));
#36820=CARTESIAN_POINT('Ctrl Pts',(0.126190709303508,-0.0355990566133874,
10.6801818582265));
#36821=CARTESIAN_POINT('Ctrl Pts',(0.113106530347436,-0.0641959568676066,
10.6646713825649));
#36822=CARTESIAN_POINT('Ctrl Pts',(0.104130112732119,-0.0751729867880824,
10.6544069799274));
#36823=CARTESIAN_POINT('Ctrl Pts',(0.0846768485015844,-0.0912869792271854,
10.6336828384074));
#36824=CARTESIAN_POINT('Ctrl Pts',(0.0730376318384033,-0.097038691048342,
10.6218026292622));
#36825=CARTESIAN_POINT('Ctrl Pts',(0.0540917217987876,-0.101964920739599,
10.6056067063421));
#36826=CARTESIAN_POINT('Ctrl Pts',(0.0476893855684835,-0.103106895932074,
10.6004594386308));
#36827=CARTESIAN_POINT('Ctrl Pts',(0.0399999999999999,-0.103841838612921,
10.5955522523606));
#36828=CARTESIAN_POINT('Origin',(0.04,0.,10.58));
#36829=CARTESIAN_POINT('',(0.0399999999999996,-0.105,10.58));
#36830=CARTESIAN_POINT('Origin',(0.04,0.,10.58));
#36831=CARTESIAN_POINT('',(0.245,-0.105,10.58));
#36832=CARTESIAN_POINT('Origin',(0.04,0.,10.58));
#36833=CARTESIAN_POINT('Ctrl Pts',(0.00894444267269635,0.0995991814488194,
10.6458389285088));
#36834=CARTESIAN_POINT('Ctrl Pts',(0.0132379567575632,0.0992136050812441,
10.6483379094571));
#36835=CARTESIAN_POINT('Ctrl Pts',(0.0183531529868693,0.0984395024940475,
10.6518751113904));
#36836=CARTESIAN_POINT('Ctrl Pts',(0.0347076968180254,0.0945110273189231,
10.6639299928277));
#36837=CARTESIAN_POINT('Ctrl Pts',(0.0471226277111957,0.0892804802504122,
10.6739642355804));
#36838=CARTESIAN_POINT('Ctrl Pts',(0.0685122659420266,0.0739398403060646,
10.6909132508036));
#36839=CARTESIAN_POINT('Ctrl Pts',(0.0790926347687259,0.0632798166374917,
10.6991949609786));
#36840=CARTESIAN_POINT('Ctrl Pts',(0.095041784574442,0.0352045494840137,
10.7113488867527));
#36841=CARTESIAN_POINT('Ctrl Pts',(0.104990250453808,-1.94764728236301E-14,
10.7186701978954));
#36842=CARTESIAN_POINT('Ctrl Pts',(0.0950417845744413,-0.0352045494840311,
10.7113488867527));
#36843=CARTESIAN_POINT('Ctrl Pts',(0.0790926347687328,-0.0632798166374956,
10.6991949609786));
#36844=CARTESIAN_POINT('Ctrl Pts',(0.0685122659420257,-0.0739398403060731,
10.6909132508036));
#36845=CARTESIAN_POINT('Ctrl Pts',(0.047122627711224,-0.0892804802503985,
10.6739642355805));
#36846=CARTESIAN_POINT('Ctrl Pts',(0.0347076968180293,-0.0945110273189234,
10.6639299928277));
#36847=CARTESIAN_POINT('Ctrl Pts',(0.0183531529868686,-0.0984395024940474,
10.6518751113904));
#36848=CARTESIAN_POINT('Ctrl Pts',(0.0132379567575637,-0.099213605081244,
10.6483379094571));
#36849=CARTESIAN_POINT('Ctrl Pts',(0.00894444267269703,-0.0995991814488193,
10.6458389285088));
#36850=CARTESIAN_POINT('Ctrl Pts',(0.0192962951151303,0.10101340050352,
10.6290767031261));
#36851=CARTESIAN_POINT('Ctrl Pts',(0.0246829710160882,0.100510889482336,
10.6323644063093));
#36852=CARTESIAN_POINT('Ctrl Pts',(0.0302700623455481,0.0996151368283168,
10.636456666124));
#36853=CARTESIAN_POINT('Ctrl Pts',(0.0474468559781996,0.0953527264698026,
10.6498673135763));
#36854=CARTESIAN_POINT('Ctrl Pts',(0.0596224855482002,0.0899496672599846,
10.6605286913046));
#36855=CARTESIAN_POINT('Ctrl Pts',(0.0803741298379308,0.0743507178323205,
10.6787417409477));
#36856=CARTESIAN_POINT('Ctrl Pts',(0.0904178647965569,0.0635857671411624,
10.6876757555526));
#36857=CARTESIAN_POINT('Ctrl Pts',(0.105408337598459,0.0353360773731678,
10.7009599149888));
#36858=CARTESIAN_POINT('Ctrl Pts',(0.114618845129398,-1.94606231903746E-14,
10.7090623931681));
#36859=CARTESIAN_POINT('Ctrl Pts',(0.105408337598459,-0.0353360773731852,
10.7009599149888));
#36860=CARTESIAN_POINT('Ctrl Pts',(0.0904178647965638,-0.0635857671411668,
10.6876757555526));
#36861=CARTESIAN_POINT('Ctrl Pts',(0.08037412983793,-0.074350717832329,
10.6787417409477));
#36862=CARTESIAN_POINT('Ctrl Pts',(0.0596224855482286,-0.0899496672599712,
10.6605286913046));
#36863=CARTESIAN_POINT('Ctrl Pts',(0.0474468559782033,-0.0953527264698027,
10.6498673135763));
#36864=CARTESIAN_POINT('Ctrl Pts',(0.0302700623455475,-0.0996151368283167,
10.636456666124));
#36865=CARTESIAN_POINT('Ctrl Pts',(0.0246829710160884,-0.100510889482335,
10.6323644063093));
#36866=CARTESIAN_POINT('Ctrl Pts',(0.0192962951151313,-0.10101340050352,
10.6290767031261));
#36867=CARTESIAN_POINT('Ctrl Pts',(0.0296481475575642,0.102427619558221,
10.6123144777433));
#36868=CARTESIAN_POINT('Ctrl Pts',(0.0362443713099573,0.101809611530983,
10.6164329417787));
#36869=CARTESIAN_POINT('Ctrl Pts',(0.0421748124401054,0.100789286405329,
10.6210251516086));
#36870=CARTESIAN_POINT('Ctrl Pts',(0.0602984726782332,0.0961969918974622,
10.6358653085135));
#36871=CARTESIAN_POINT('Ctrl Pts',(0.0721769906646143,0.0906177922175886,
10.6471183826832));
#36872=CARTESIAN_POINT('Ctrl Pts',(0.0922682488362055,0.0747621092618343,
10.6665784897832));
#36873=CARTESIAN_POINT('Ctrl Pts',(0.101781300319608,0.0638900063639316,
10.6761905879909));
#36874=CARTESIAN_POINT('Ctrl Pts',(0.115824156279493,0.0354675287242178,
10.6905708299903));
#36875=CARTESIAN_POINT('Ctrl Pts',(0.12429176962826,-1.94491199561677E-14,
10.6994790798386));
#36876=CARTESIAN_POINT('Ctrl Pts',(0.115824156279491,-0.0354675287242332,
10.6905708299903));
#36877=CARTESIAN_POINT('Ctrl Pts',(0.101781300319605,-0.0638900063639355,
10.6761905879909));
#36878=CARTESIAN_POINT('Ctrl Pts',(0.0922682488362152,-0.0747621092618265,
10.6665784897832));
#36879=CARTESIAN_POINT('Ctrl Pts',(0.0721769906645798,-0.0906177922176127,
10.6471183826832));
#36880=CARTESIAN_POINT('Ctrl Pts',(0.0602984726782293,-0.0961969918974626,
10.6358653085135));
#36881=CARTESIAN_POINT('Ctrl Pts',(0.0421748124401086,-0.100789286405329,
10.6210251516086));
#36882=CARTESIAN_POINT('Ctrl Pts',(0.0362443713099588,-0.101809611530983,
10.6164329417787));
#36883=CARTESIAN_POINT('Ctrl Pts',(0.0296481475575656,-0.102427619558221,
10.6123144777433));
#36884=CARTESIAN_POINT('Ctrl Pts',(0.0399999999999981,0.103841838612921,
10.5955522523606));
#36885=CARTESIAN_POINT('Ctrl Pts',(0.0476893855684824,0.103106895932074,
10.6004594386308));
#36886=CARTESIAN_POINT('Ctrl Pts',(0.0540917217987843,0.101964920739599,
10.6056067063421));
#36887=CARTESIAN_POINT('Ctrl Pts',(0.0730376318384075,0.0970386910483417,
10.6218026292622));
#36888=CARTESIAN_POINT('Ctrl Pts',(0.0846768485016188,0.0912869792271611,
10.6336828384074));
#36889=CARTESIAN_POINT('Ctrl Pts',(0.10413011273211,0.0751729867880902,
10.6544069799274));
#36890=CARTESIAN_POINT('Ctrl Pts',(0.113106530347439,0.0641959568676023,
10.6646713825649));
#36891=CARTESIAN_POINT('Ctrl Pts',(0.12619070930351,0.0355990566133719,
10.6801818582265));
#36892=CARTESIAN_POINT('Ctrl Pts',(0.13392036430385,-1.94332703229122E-14,
10.6898712751113));
#36893=CARTESIAN_POINT('Ctrl Pts',(0.126190709303508,-0.0355990566133874,
10.6801818582265));
#36894=CARTESIAN_POINT('Ctrl Pts',(0.113106530347436,-0.0641959568676066,
10.6646713825649));
#36895=CARTESIAN_POINT('Ctrl Pts',(0.104130112732119,-0.0751729867880824,
10.6544069799274));
#36896=CARTESIAN_POINT('Ctrl Pts',(0.0846768485015844,-0.0912869792271854,
10.6336828384074));
#36897=CARTESIAN_POINT('Ctrl Pts',(0.0730376318384033,-0.097038691048342,
10.6218026292622));
#36898=CARTESIAN_POINT('Ctrl Pts',(0.0540917217987876,-0.101964920739599,
10.6056067063421));
#36899=CARTESIAN_POINT('Ctrl Pts',(0.0476893855684835,-0.103106895932074,
10.6004594386308));
#36900=CARTESIAN_POINT('Ctrl Pts',(0.0399999999999999,-0.103841838612921,
10.5955522523606));
#36901=CARTESIAN_POINT('Ctrl Pts',(0.04,0.103841838612921,10.5955522523606));
#36902=CARTESIAN_POINT('Ctrl Pts',(0.04,0.102606878649513,10.6075587254027));
#36903=CARTESIAN_POINT('Ctrl Pts',(0.0399999999999975,0.101164195082993,
10.6196695728954));
#36904=CARTESIAN_POINT('Ctrl Pts',(0.0399999999999975,0.0972792927935932,
10.6440647058907));
#36905=CARTESIAN_POINT('Ctrl Pts',(0.04,0.0948285697695771,10.6562661891283));
#36906=CARTESIAN_POINT('Ctrl Pts',(0.04,0.0916515138991168,10.6683225406115));
#36907=CARTESIAN_POINT('Ctrl Pts',(0.04,-0.0916515138991168,10.6683225406115));
#36908=CARTESIAN_POINT('Ctrl Pts',(0.04,-0.0935748723716089,10.6610237436378));
#36909=CARTESIAN_POINT('Ctrl Pts',(0.0399999999895056,-0.0952353918400671,
10.6536541522208));
#36910=CARTESIAN_POINT('Ctrl Pts',(0.0399999999895056,-0.0999669573193089,
10.62939385374));
#36911=CARTESIAN_POINT('Ctrl Pts',(0.0400000000000004,-0.102095272100589,
10.6125326439262));
#36912=CARTESIAN_POINT('Ctrl Pts',(0.0400000000000004,-0.103841838612921,
10.5955522523606));
#36913=CARTESIAN_POINT('Origin',(0.55,0.,10.725));
#36914=CARTESIAN_POINT('',(0.435,1.40834381901946E-17,10.71));
#36915=CARTESIAN_POINT('Origin',(0.55,0.,10.71));
#36916=CARTESIAN_POINT('',(0.465,-1.04094977927525E-17,10.74));
#36917=CARTESIAN_POINT('',(0.45,1.22464679914735E-17,10.725));
#36918=CARTESIAN_POINT('Origin',(0.55,0.,10.74));
#36919=CARTESIAN_POINT('Origin',(0.55,0.,10.825));
#36920=CARTESIAN_POINT('',(0.465,1.04094977927525E-17,10.88));
#36921=CARTESIAN_POINT('',(0.465,-1.04094977927525E-17,10.825));
#36922=CARTESIAN_POINT('Origin',(0.55,0.,10.88));
#36923=CARTESIAN_POINT('Origin',(0.7,0.,10.71));
#36924=CARTESIAN_POINT('',(0.68,8.327598234202E-17,10.71));
#36925=CARTESIAN_POINT('Origin',(0.,0.,10.71));
#36926=CARTESIAN_POINT('',(-0.39,0.476313972081441,10.71));
#36927=CARTESIAN_POINT('Origin',(-0.275,0.476313972081441,10.71));
#36928=CARTESIAN_POINT('',(-0.39,-0.476313972081441,10.71));
#36929=CARTESIAN_POINT('Origin',(-0.275,-0.476313972081441,10.71));
#36930=CARTESIAN_POINT('Origin',(0.55,0.,10.895));
#36931=CARTESIAN_POINT('',(0.435,-1.40834381901946E-17,10.91));
#36932=CARTESIAN_POINT('Origin',(0.55,0.,10.91));
#36933=CARTESIAN_POINT('',(0.45,-1.22464679914735E-17,10.895));
#36934=CARTESIAN_POINT('Origin',(0.2,0.,10.91));
#36935=CARTESIAN_POINT('',(0.68,-8.327598234202E-17,10.91));
#36936=CARTESIAN_POINT('Origin',(0.,0.,10.91));
#36937=CARTESIAN_POINT('',(-0.39,0.476313972081441,10.91));
#36938=CARTESIAN_POINT('Origin',(-0.275,0.476313972081441,10.91));
#36939=CARTESIAN_POINT('',(-0.39,-0.476313972081441,10.91));
#36940=CARTESIAN_POINT('Origin',(-0.275,-0.476313972081441,10.91));
#36941=CARTESIAN_POINT('Origin',(-0.275,0.476313972081441,10.725));
#36942=CARTESIAN_POINT('',(-0.36,0.476313972081441,10.74));
#36943=CARTESIAN_POINT('',(-0.375,0.476313972081441,10.725));
#36944=CARTESIAN_POINT('Origin',(-0.275,0.476313972081441,10.74));
#36945=CARTESIAN_POINT('Origin',(-0.275,0.476313972081441,10.825));
#36946=CARTESIAN_POINT('',(-0.36,0.476313972081441,10.88));
#36947=CARTESIAN_POINT('',(-0.36,0.476313972081441,10.825));
#36948=CARTESIAN_POINT('Origin',(-0.275,0.476313972081441,10.88));
#36949=CARTESIAN_POINT('Origin',(-0.275,0.476313972081441,10.895));
#36950=CARTESIAN_POINT('',(-0.375,0.476313972081441,10.895));
#36951=CARTESIAN_POINT('Origin',(-0.275,-0.476313972081441,10.725));
#36952=CARTESIAN_POINT('',(-0.36,-0.476313972081441,10.74));
#36953=CARTESIAN_POINT('',(-0.375,-0.476313972081441,10.725));
#36954=CARTESIAN_POINT('Origin',(-0.275,-0.476313972081441,10.74));
#36955=CARTESIAN_POINT('Origin',(-0.275,-0.476313972081441,10.825));
#36956=CARTESIAN_POINT('',(-0.36,-0.476313972081441,10.88));
#36957=CARTESIAN_POINT('',(-0.36,-0.476313972081441,10.825));
#36958=CARTESIAN_POINT('Origin',(-0.275,-0.476313972081441,10.88));
#36959=CARTESIAN_POINT('Origin',(-0.275,-0.476313972081441,10.895));
#36960=CARTESIAN_POINT('',(-0.375,-0.476313972081441,10.895));
#36961=CARTESIAN_POINT('Origin',(0.04,0.105,10.58));
#36962=CARTESIAN_POINT('Origin',(0.04,0.105,10.58));
#36963=CARTESIAN_POINT('Origin',(0.,0.,10.9));
#36964=CARTESIAN_POINT('',(0.7,8.57252759403147E-17,10.89));
#36965=CARTESIAN_POINT('',(0.69,8.45006291411674E-17,10.9));
#36966=CARTESIAN_POINT('',(-0.7,-8.57252759403147E-17,10.89));
#36967=CARTESIAN_POINT('Origin',(0.,0.,10.89));
#36968=CARTESIAN_POINT('Origin',(0.,0.,10.89));
#36969=CARTESIAN_POINT('Origin',(0.,0.,10.81));
#36970=CARTESIAN_POINT('',(-0.7,-8.57252759403147E-17,10.73));
#36971=CARTESIAN_POINT('',(-0.7,-8.57252759403147E-17,10.81));
#36972=CARTESIAN_POINT('',(0.7,-8.57252759403147E-17,10.73));
#36973=CARTESIAN_POINT('Origin',(0.,0.,10.73));
#36974=CARTESIAN_POINT('Origin',(0.,0.,10.73));
#36975=CARTESIAN_POINT('Origin',(0.,0.,10.72));
#36976=CARTESIAN_POINT('',(0.69,8.45006291411674E-17,10.72));
#54967=UNCERTAINTY_MEASURE_WITH_UNIT(LENGTH_MEASURE(0.001),#55003,
'DISTANCE_ACCURACY_VALUE',
'Maximum model space distance between geometric entities at asserted c
onnectivities');
#54980=UNCERTAINTY_MEASURE_WITH_UNIT(LENGTH_MEASURE(0.001),#55003,
'DISTANCE_ACCURACY_VALUE',
'Maximum model space distance between geometric entities at asserted c
onnectivities');
#54989=(
GEOMETRIC_REPRESENTATION_CONTEXT(3)
GLOBAL_UNCERTAINTY_ASSIGNED_CONTEXT((#54967))
GLOBAL_UNIT_ASSIGNED_CONTEXT((#55003,#55005,#55006))
REPRESENTATION_CONTEXT('','3D')
);
#55002=(
GEOMETRIC_REPRESENTATION_CONTEXT(3)
GLOBAL_UNCERTAINTY_ASSIGNED_CONTEXT((#54980))
GLOBAL_UNIT_ASSIGNED_CONTEXT((#55003,#55005,#55006))
REPRESENTATION_CONTEXT('','3D')
);
#55003=(
LENGTH_UNIT()
NAMED_UNIT(*)
SI_UNIT(.CENTI.,.METRE.)
);
#55005=(
NAMED_UNIT(*)
PLANE_ANGLE_UNIT()
SI_UNIT($,.RADIAN.)
);
#55006=(
NAMED_UNIT(*)
SI_UNIT($,.STERADIAN.)
SOLID_ANGLE_UNIT()
);
#55015=SHAPE_DEFINITION_REPRESENTATION(#55036,#55111);
#55036=PRODUCT_DEFINITION_SHAPE('',$,#55133);
#55111=SHAPE_REPRESENTATION('',(#25845),#54989);
#55124=PRODUCT_DEFINITION_CONTEXT('part definition',#55189,'design');
#55133=PRODUCT_DEFINITION('2026-10-18-23-36-21-472',
'08_Disc_Aluminium_Hub_Clamp_Adapter',#55154,#55124);
#55154=PRODUCT_DEFINITION_FORMATION('',$,#55199);
#55189=APPLICATION_CONTEXT(
'Core Data for Automotive Mechanical Design Process');
#55190=PRODUCT_CONTEXT('part definition',#55189,'mechanical');
#55199=PRODUCT('2026-10-18-23-36-21-472',
'08_Disc_Aluminium_Hub_Clamp_Adapter',$,(#55190));
#55366=COLOUR_RGB('Light Blue',0.38,0.62,0.78);
#55367=FILL_AREA_STYLE_COLOUR('',#55366);
#55368=FILL_AREA_STYLE('',(#55367));
#55369=SURFACE_STYLE_FILL_AREA(#55368);
#55370=SURFACE_SIDE_STYLE('',(#55369));
#55371=SURFACE_STYLE_USAGE(.BOTH.,#55370);
#55372=PRESENTATION_STYLE_ASSIGNMENT((#55371));
ENDSEC;
END-ISO-10303-21;
